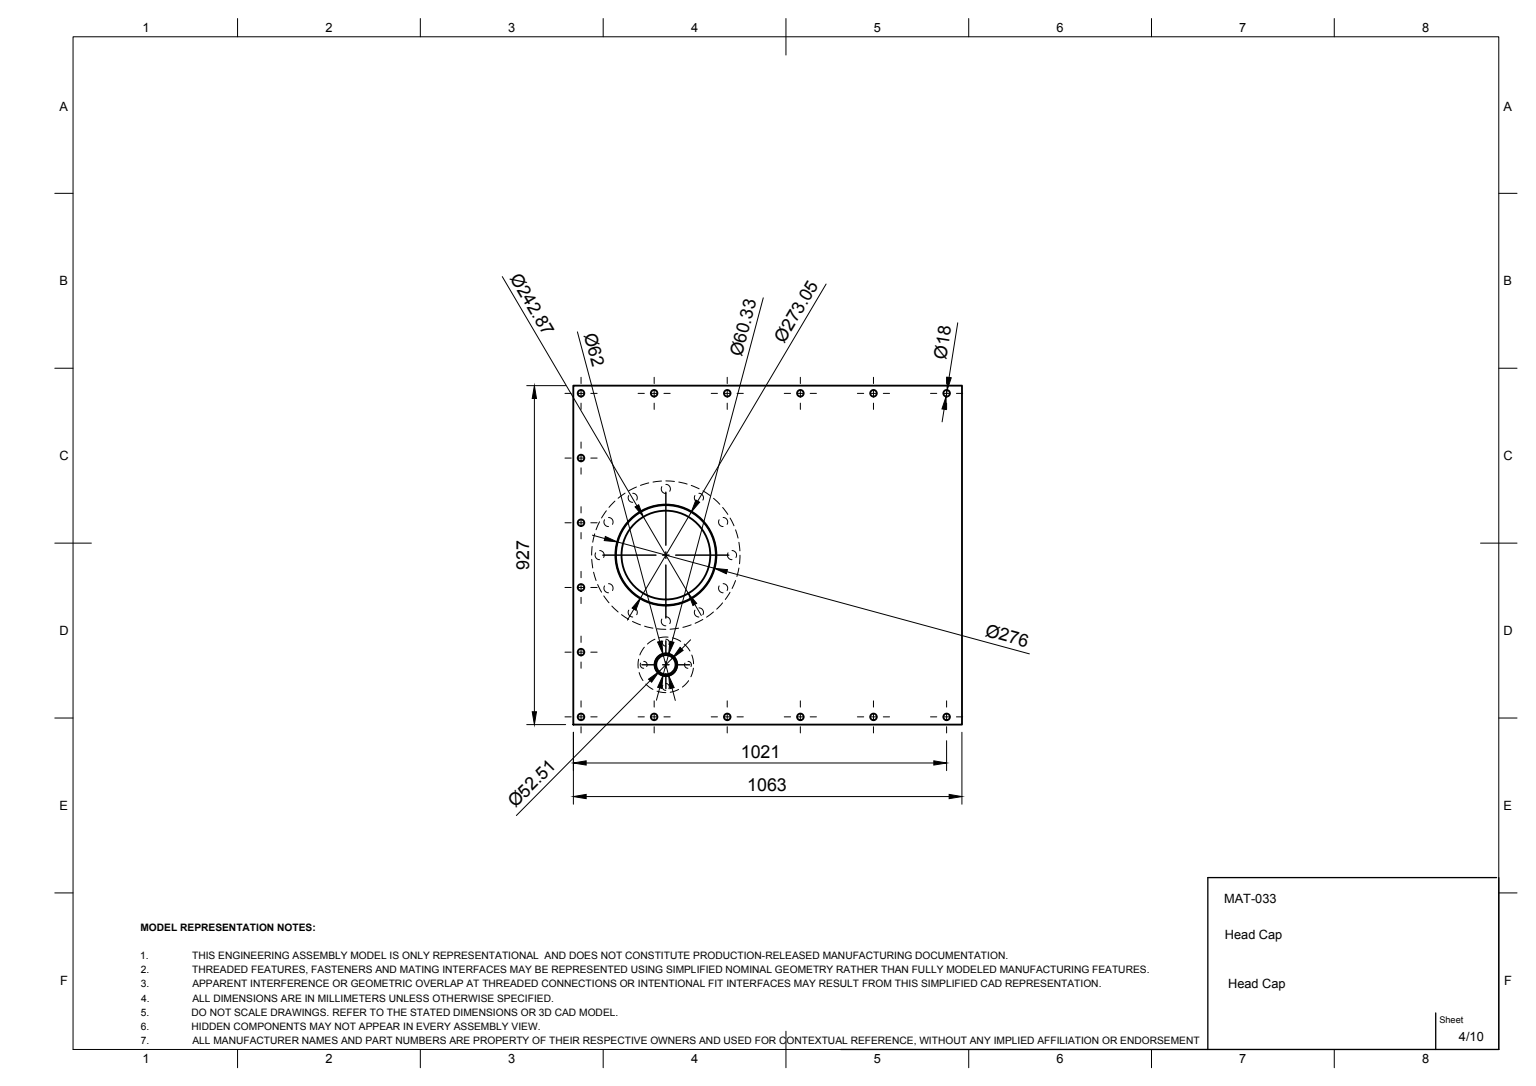
ISO-10303-21;
HEADER;
/* Generated by software containing ST-Developer
 * from STEP Tools, Inc. (www.steptools.com) 
 */

FILE_DESCRIPTION(
/* description */ ('STEP AP214'),
/* implementation_level */ '2;1');

FILE_NAME(
/* name */ 'Head Cap.step',
/* time_stamp */ '2026-11-14T07:13:32-08:00',
/* author */ (''),
/* organization */ (''),
/* preprocessor_version */ 'ST-DEVELOPER v20.2',
/* originating_system */ 'Autodesk Translation Framework v15.17.0.0',
/* authorisation */ '');

FILE_SCHEMA (('AUTOMOTIVE_DESIGN { 1 0 10303 214 3 1 1 }'));
ENDSEC;

DATA;
#10=MECHANICAL_DESIGN_GEOMETRIC_PRESENTATION_REPRESENTATION('',(#1300,#1301,#1302,#1303,#1304),#32903);
#673=SHAPE_REPRESENTATION_RELATIONSHIP('SRR','None',#33014,#687);
#687=ADVANCED_BREP_SHAPE_REPRESENTATION('',(#1389,#1390,#1391,#1392,#1393),
#32889);
#736=CIRCLE('',#15901,9.00000000000006);
#737=CIRCLE('',#15902,9.00000000000006);
#738=CIRCLE('',#15904,9.00000000000006);
#739=CIRCLE('',#15905,9.00000000000006);
#740=CIRCLE('',#15907,9.00000000000005);
#741=CIRCLE('',#15908,9.00000000000005);
#742=CIRCLE('',#15910,9.00000000000005);
#743=CIRCLE('',#15911,9.00000000000005);
#744=CIRCLE('',#15913,9.00000000000006);
#745=CIRCLE('',#15914,9.00000000000006);
#746=CIRCLE('',#15916,9.00000000000006);
#747=CIRCLE('',#15917,9.00000000000006);
#748=CIRCLE('',#15919,9.00000000000006);
#749=CIRCLE('',#15920,9.00000000000006);
#750=CIRCLE('',#15922,9.00000000000006);
#751=CIRCLE('',#15923,9.00000000000006);
#752=CIRCLE('',#15925,9.00000000000006);
#753=CIRCLE('',#15926,9.00000000000006);
#754=CIRCLE('',#15928,9.00000000000006);
#755=CIRCLE('',#15929,9.00000000000006);
#756=CIRCLE('',#15931,9.00000000000406);
#757=CIRCLE('',#15932,9.00000000000406);
#758=CIRCLE('',#15934,9.00000000000006);
#759=CIRCLE('',#15935,9.00000000000006);
#760=CIRCLE('',#15937,9.00000000000006);
#761=CIRCLE('',#15938,9.00000000000006);
#762=CIRCLE('',#15940,9.00000000000006);
#763=CIRCLE('',#15941,9.00000000000006);
#764=CIRCLE('',#15943,9.00000000000006);
#765=CIRCLE('',#15944,9.00000000000006);
#766=CIRCLE('',#15946,31.0000000000001);
#767=CIRCLE('',#15947,31.0000000000001);
#768=CIRCLE('',#15949,138.);
#769=CIRCLE('',#15950,138.);
#770=CIRCLE('',#15952,9.00000000000006);
#771=CIRCLE('',#15953,9.00000000000006);
#772=CIRCLE('',#15961,136.525);
#773=CIRCLE('',#15962,136.525);
#774=CIRCLE('',#15964,121.435);
#775=CIRCLE('',#15965,121.435);
#776=CIRCLE('',#15969,30.165);
#777=CIRCLE('',#15970,30.165);
#778=CIRCLE('',#15972,26.255);
#779=CIRCLE('',#15973,26.255);
#780=CIRCLE('',#15977,12.4999999999953);
#781=CIRCLE('',#15978,12.4999999999953);
#782=CIRCLE('',#15980,12.4999999999835);
#783=CIRCLE('',#15981,12.4999999999835);
#784=CIRCLE('',#15983,12.4999999999698);
#785=CIRCLE('',#15984,12.4999999999698);
#786=CIRCLE('',#15986,12.4999999999583);
#787=CIRCLE('',#15987,12.4999999999583);
#788=CIRCLE('',#15989,12.4999999999518);
#789=CIRCLE('',#15990,12.4999999999518);
#790=CIRCLE('',#15992,12.4999999999521);
#791=CIRCLE('',#15993,12.4999999999521);
#792=CIRCLE('',#15995,12.499999999959);
#793=CIRCLE('',#15996,12.499999999959);
#794=CIRCLE('',#15998,12.4999999999705);
#795=CIRCLE('',#15999,12.4999999999705);
#796=CIRCLE('',#16001,12.4999999999835);
#797=CIRCLE('',#16002,12.4999999999835);
#798=CIRCLE('',#16004,12.4999999999946);
#799=CIRCLE('',#16005,12.4999999999946);
#800=CIRCLE('',#16007,12.5000000000006);
#801=CIRCLE('',#16008,12.5000000000006);
#802=CIRCLE('',#16010,12.5);
#803=CIRCLE('',#16011,12.5);
#804=CIRCLE('',#16013,138.);
#805=CIRCLE('',#16014,138.);
#806=CIRCLE('',#16016,203.);
#807=CIRCLE('',#16017,203.);
#808=CIRCLE('',#16021,9.50000000000001);
#809=CIRCLE('',#16022,9.50000000000001);
#810=CIRCLE('',#16024,9.50000000000006);
#811=CIRCLE('',#16025,9.50000000000006);
#812=CIRCLE('',#16027,9.50000000000001);
#813=CIRCLE('',#16028,9.49999999999998);
#814=CIRCLE('',#16030,9.50000000000001);
#815=CIRCLE('',#16031,9.50000000000001);
#816=CIRCLE('',#16033,31.);
#817=CIRCLE('',#16034,31.);
#818=CIRCLE('',#16036,76.0000000000001);
#819=CIRCLE('',#16037,76.0000000000001);
#1099=CYLINDRICAL_SURFACE('',#15900,9.00000000000006);
#1100=CYLINDRICAL_SURFACE('',#15903,9.00000000000006);
#1101=CYLINDRICAL_SURFACE('',#15906,9.00000000000005);
#1102=CYLINDRICAL_SURFACE('',#15909,9.00000000000005);
#1103=CYLINDRICAL_SURFACE('',#15912,9.00000000000006);
#1104=CYLINDRICAL_SURFACE('',#15915,9.00000000000006);
#1105=CYLINDRICAL_SURFACE('',#15918,9.00000000000006);
#1106=CYLINDRICAL_SURFACE('',#15921,9.00000000000006);
#1107=CYLINDRICAL_SURFACE('',#15924,9.00000000000006);
#1108=CYLINDRICAL_SURFACE('',#15927,9.00000000000006);
#1109=CYLINDRICAL_SURFACE('',#15930,9.00000000000406);
#1110=CYLINDRICAL_SURFACE('',#15933,9.00000000000006);
#1111=CYLINDRICAL_SURFACE('',#15936,9.00000000000006);
#1112=CYLINDRICAL_SURFACE('',#15939,9.00000000000006);
#1113=CYLINDRICAL_SURFACE('',#15942,9.00000000000006);
#1114=CYLINDRICAL_SURFACE('',#15945,31.0000000000001);
#1115=CYLINDRICAL_SURFACE('',#15948,138.);
#1116=CYLINDRICAL_SURFACE('',#15951,9.00000000000006);
#1117=CYLINDRICAL_SURFACE('',#15960,136.525);
#1118=CYLINDRICAL_SURFACE('',#15963,121.435);
#1119=CYLINDRICAL_SURFACE('',#15968,30.165);
#1120=CYLINDRICAL_SURFACE('',#15971,26.255);
#1121=CYLINDRICAL_SURFACE('',#15976,12.4999999999953);
#1122=CYLINDRICAL_SURFACE('',#15979,12.4999999999835);
#1123=CYLINDRICAL_SURFACE('',#15982,12.4999999999698);
#1124=CYLINDRICAL_SURFACE('',#15985,12.4999999999583);
#1125=CYLINDRICAL_SURFACE('',#15988,12.4999999999518);
#1126=CYLINDRICAL_SURFACE('',#15991,12.4999999999521);
#1127=CYLINDRICAL_SURFACE('',#15994,12.499999999959);
#1128=CYLINDRICAL_SURFACE('',#15997,12.4999999999705);
#1129=CYLINDRICAL_SURFACE('',#16000,12.4999999999835);
#1130=CYLINDRICAL_SURFACE('',#16003,12.4999999999946);
#1131=CYLINDRICAL_SURFACE('',#16006,12.5000000000006);
#1132=CYLINDRICAL_SURFACE('',#16009,12.5);
#1133=CYLINDRICAL_SURFACE('',#16012,138.);
#1134=CYLINDRICAL_SURFACE('',#16015,203.);
#1135=CYLINDRICAL_SURFACE('',#16020,9.50000000000001);
#1136=CYLINDRICAL_SURFACE('',#16023,9.50000000000006);
#1137=CYLINDRICAL_SURFACE('',#16026,9.50000000000001);
#1138=CYLINDRICAL_SURFACE('',#16029,9.50000000000001);
#1139=CYLINDRICAL_SURFACE('',#16032,31.);
#1140=CYLINDRICAL_SURFACE('',#16035,76.0000000000001);
#1300=STYLED_ITEM('',(#33097),#1389);
#1301=STYLED_ITEM('',(#33097),#1390);
#1302=STYLED_ITEM('',(#33097),#1391);
#1303=STYLED_ITEM('',(#33097),#1392);
#1304=STYLED_ITEM('',(#33097),#1393);
#1389=MANIFOLD_SOLID_BREP('Body1',#15548);
#1390=MANIFOLD_SOLID_BREP('Body2',#15549);
#1391=MANIFOLD_SOLID_BREP('Body3',#15550);
#1392=MANIFOLD_SOLID_BREP('Body4',#15551);
#1393=MANIFOLD_SOLID_BREP('Body5',#15552);
#1503=FACE_BOUND('',#2706,.T.);
#1504=FACE_BOUND('',#2707,.T.);
#1505=FACE_BOUND('',#2708,.T.);
#1506=FACE_BOUND('',#2709,.T.);
#1507=FACE_BOUND('',#2710,.T.);
#1508=FACE_BOUND('',#2711,.T.);
#1509=FACE_BOUND('',#2712,.T.);
#1510=FACE_BOUND('',#2713,.T.);
#1511=FACE_BOUND('',#2714,.T.);
#1512=FACE_BOUND('',#2715,.T.);
#1513=FACE_BOUND('',#2716,.T.);
#1514=FACE_BOUND('',#2717,.T.);
#1515=FACE_BOUND('',#2718,.T.);
#1516=FACE_BOUND('',#2719,.T.);
#1517=FACE_BOUND('',#2720,.T.);
#1518=FACE_BOUND('',#2721,.T.);
#1519=FACE_BOUND('',#2722,.T.);
#1520=FACE_BOUND('',#2723,.T.);
#1521=FACE_BOUND('',#2725,.T.);
#1522=FACE_BOUND('',#2726,.T.);
#1523=FACE_BOUND('',#2727,.T.);
#1524=FACE_BOUND('',#2728,.T.);
#1525=FACE_BOUND('',#2729,.T.);
#1526=FACE_BOUND('',#2730,.T.);
#1527=FACE_BOUND('',#2731,.T.);
#1528=FACE_BOUND('',#2732,.T.);
#1529=FACE_BOUND('',#2733,.T.);
#1530=FACE_BOUND('',#2734,.T.);
#1531=FACE_BOUND('',#2735,.T.);
#1532=FACE_BOUND('',#2736,.T.);
#1533=FACE_BOUND('',#2737,.T.);
#1534=FACE_BOUND('',#2738,.T.);
#1535=FACE_BOUND('',#2739,.T.);
#1536=FACE_BOUND('',#2740,.T.);
#1537=FACE_BOUND('',#2741,.T.);
#1538=FACE_BOUND('',#2742,.T.);
#1539=FACE_BOUND('',#2746,.T.);
#1540=FACE_BOUND('',#2748,.T.);
#1541=FACE_BOUND('',#2752,.T.);
#1542=FACE_BOUND('',#2754,.T.);
#1543=FACE_BOUND('',#2770,.T.);
#1544=FACE_BOUND('',#2771,.T.);
#1545=FACE_BOUND('',#2772,.T.);
#1546=FACE_BOUND('',#2773,.T.);
#1547=FACE_BOUND('',#2774,.T.);
#1548=FACE_BOUND('',#2775,.T.);
#1549=FACE_BOUND('',#2776,.T.);
#1550=FACE_BOUND('',#2777,.T.);
#1551=FACE_BOUND('',#2778,.T.);
#1552=FACE_BOUND('',#2779,.T.);
#1553=FACE_BOUND('',#2780,.T.);
#1554=FACE_BOUND('',#2781,.T.);
#1555=FACE_BOUND('',#2782,.T.);
#1556=FACE_BOUND('',#2784,.T.);
#1557=FACE_BOUND('',#2785,.T.);
#1558=FACE_BOUND('',#2786,.T.);
#1559=FACE_BOUND('',#2787,.T.);
#1560=FACE_BOUND('',#2788,.T.);
#1561=FACE_BOUND('',#2789,.T.);
#1562=FACE_BOUND('',#2790,.T.);
#1563=FACE_BOUND('',#2791,.T.);
#1564=FACE_BOUND('',#2792,.T.);
#1565=FACE_BOUND('',#2793,.T.);
#1566=FACE_BOUND('',#2794,.T.);
#1567=FACE_BOUND('',#2795,.T.);
#1568=FACE_BOUND('',#2796,.T.);
#1569=FACE_BOUND('',#2804,.T.);
#1570=FACE_BOUND('',#2805,.T.);
#1571=FACE_BOUND('',#2806,.T.);
#1572=FACE_BOUND('',#2807,.T.);
#1573=FACE_BOUND('',#2808,.T.);
#1574=FACE_BOUND('',#2810,.T.);
#1575=FACE_BOUND('',#2811,.T.);
#1576=FACE_BOUND('',#2812,.T.);
#1577=FACE_BOUND('',#2813,.T.);
#1578=FACE_BOUND('',#2814,.T.);
#1754=FACE_OUTER_BOUND('',#2683,.T.);
#1755=FACE_OUTER_BOUND('',#2684,.T.);
#1756=FACE_OUTER_BOUND('',#2685,.T.);
#1757=FACE_OUTER_BOUND('',#2686,.T.);
#1758=FACE_OUTER_BOUND('',#2687,.T.);
#1759=FACE_OUTER_BOUND('',#2688,.T.);
#1760=FACE_OUTER_BOUND('',#2689,.T.);
#1761=FACE_OUTER_BOUND('',#2690,.T.);
#1762=FACE_OUTER_BOUND('',#2691,.T.);
#1763=FACE_OUTER_BOUND('',#2692,.T.);
#1764=FACE_OUTER_BOUND('',#2693,.T.);
#1765=FACE_OUTER_BOUND('',#2694,.T.);
#1766=FACE_OUTER_BOUND('',#2695,.T.);
#1767=FACE_OUTER_BOUND('',#2696,.T.);
#1768=FACE_OUTER_BOUND('',#2697,.T.);
#1769=FACE_OUTER_BOUND('',#2698,.T.);
#1770=FACE_OUTER_BOUND('',#2699,.T.);
#1771=FACE_OUTER_BOUND('',#2700,.T.);
#1772=FACE_OUTER_BOUND('',#2701,.T.);
#1773=FACE_OUTER_BOUND('',#2702,.T.);
#1774=FACE_OUTER_BOUND('',#2703,.T.);
#1775=FACE_OUTER_BOUND('',#2704,.T.);
#1776=FACE_OUTER_BOUND('',#2705,.T.);
#1777=FACE_OUTER_BOUND('',#2724,.T.);
#1778=FACE_OUTER_BOUND('',#2743,.T.);
#1779=FACE_OUTER_BOUND('',#2744,.T.);
#1780=FACE_OUTER_BOUND('',#2745,.T.);
#1781=FACE_OUTER_BOUND('',#2747,.T.);
#1782=FACE_OUTER_BOUND('',#2749,.T.);
#1783=FACE_OUTER_BOUND('',#2750,.T.);
#1784=FACE_OUTER_BOUND('',#2751,.T.);
#1785=FACE_OUTER_BOUND('',#2753,.T.);
#1786=FACE_OUTER_BOUND('',#2755,.T.);
#1787=FACE_OUTER_BOUND('',#2756,.T.);
#1788=FACE_OUTER_BOUND('',#2757,.T.);
#1789=FACE_OUTER_BOUND('',#2758,.T.);
#1790=FACE_OUTER_BOUND('',#2759,.T.);
#1791=FACE_OUTER_BOUND('',#2760,.T.);
#1792=FACE_OUTER_BOUND('',#2761,.T.);
#1793=FACE_OUTER_BOUND('',#2762,.T.);
#1794=FACE_OUTER_BOUND('',#2763,.T.);
#1795=FACE_OUTER_BOUND('',#2764,.T.);
#1796=FACE_OUTER_BOUND('',#2765,.T.);
#1797=FACE_OUTER_BOUND('',#2766,.T.);
#1798=FACE_OUTER_BOUND('',#2767,.T.);
#1799=FACE_OUTER_BOUND('',#2768,.T.);
#1800=FACE_OUTER_BOUND('',#2769,.T.);
#1801=FACE_OUTER_BOUND('',#2783,.T.);
#1802=FACE_OUTER_BOUND('',#2797,.T.);
#1803=FACE_OUTER_BOUND('',#2798,.T.);
#1804=FACE_OUTER_BOUND('',#2799,.T.);
#1805=FACE_OUTER_BOUND('',#2800,.T.);
#1806=FACE_OUTER_BOUND('',#2801,.T.);
#1807=FACE_OUTER_BOUND('',#2802,.T.);
#1808=FACE_OUTER_BOUND('',#2803,.T.);
#1809=FACE_OUTER_BOUND('',#2809,.T.);
#2683=EDGE_LOOP('',(#10267,#10268,#10269,#10270));
#2684=EDGE_LOOP('',(#10271,#10272,#10273,#10274));
#2685=EDGE_LOOP('',(#10275,#10276,#10277,#10278));
#2686=EDGE_LOOP('',(#10279,#10280,#10281,#10282));
#2687=EDGE_LOOP('',(#10283,#10284,#10285,#10286));
#2688=EDGE_LOOP('',(#10287,#10288,#10289,#10290));
#2689=EDGE_LOOP('',(#10291,#10292,#10293,#10294));
#2690=EDGE_LOOP('',(#10295,#10296,#10297,#10298));
#2691=EDGE_LOOP('',(#10299,#10300,#10301,#10302));
#2692=EDGE_LOOP('',(#10303,#10304,#10305,#10306));
#2693=EDGE_LOOP('',(#10307,#10308,#10309,#10310));
#2694=EDGE_LOOP('',(#10311,#10312,#10313,#10314));
#2695=EDGE_LOOP('',(#10315,#10316,#10317,#10318));
#2696=EDGE_LOOP('',(#10319,#10320,#10321,#10322));
#2697=EDGE_LOOP('',(#10323,#10324,#10325,#10326));
#2698=EDGE_LOOP('',(#10327,#10328,#10329,#10330));
#2699=EDGE_LOOP('',(#10331,#10332,#10333,#10334));
#2700=EDGE_LOOP('',(#10335,#10336,#10337,#10338));
#2701=EDGE_LOOP('',(#10339,#10340,#10341,#10342));
#2702=EDGE_LOOP('',(#10343,#10344,#10345,#10346));
#2703=EDGE_LOOP('',(#10347,#10348,#10349,#10350));
#2704=EDGE_LOOP('',(#10351,#10352,#10353,#10354));
#2705=EDGE_LOOP('',(#10355,#10356,#10357,#10358));
#2706=EDGE_LOOP('',(#10359));
#2707=EDGE_LOOP('',(#10360));
#2708=EDGE_LOOP('',(#10361));
#2709=EDGE_LOOP('',(#10362));
#2710=EDGE_LOOP('',(#10363));
#2711=EDGE_LOOP('',(#10364));
#2712=EDGE_LOOP('',(#10365));
#2713=EDGE_LOOP('',(#10366));
#2714=EDGE_LOOP('',(#10367));
#2715=EDGE_LOOP('',(#10368));
#2716=EDGE_LOOP('',(#10369));
#2717=EDGE_LOOP('',(#10370));
#2718=EDGE_LOOP('',(#10371));
#2719=EDGE_LOOP('',(#10372));
#2720=EDGE_LOOP('',(#10373));
#2721=EDGE_LOOP('',(#10374));
#2722=EDGE_LOOP('',(#10375));
#2723=EDGE_LOOP('',(#10376));
#2724=EDGE_LOOP('',(#10377,#10378,#10379,#10380));
#2725=EDGE_LOOP('',(#10381));
#2726=EDGE_LOOP('',(#10382));
#2727=EDGE_LOOP('',(#10383));
#2728=EDGE_LOOP('',(#10384));
#2729=EDGE_LOOP('',(#10385));
#2730=EDGE_LOOP('',(#10386));
#2731=EDGE_LOOP('',(#10387));
#2732=EDGE_LOOP('',(#10388));
#2733=EDGE_LOOP('',(#10389));
#2734=EDGE_LOOP('',(#10390));
#2735=EDGE_LOOP('',(#10391));
#2736=EDGE_LOOP('',(#10392));
#2737=EDGE_LOOP('',(#10393));
#2738=EDGE_LOOP('',(#10394));
#2739=EDGE_LOOP('',(#10395));
#2740=EDGE_LOOP('',(#10396));
#2741=EDGE_LOOP('',(#10397));
#2742=EDGE_LOOP('',(#10398));
#2743=EDGE_LOOP('',(#10399,#10400,#10401,#10402));
#2744=EDGE_LOOP('',(#10403,#10404,#10405,#10406));
#2745=EDGE_LOOP('',(#10407));
#2746=EDGE_LOOP('',(#10408));
#2747=EDGE_LOOP('',(#10409));
#2748=EDGE_LOOP('',(#10410));
#2749=EDGE_LOOP('',(#10411,#10412,#10413,#10414));
#2750=EDGE_LOOP('',(#10415,#10416,#10417,#10418));
#2751=EDGE_LOOP('',(#10419));
#2752=EDGE_LOOP('',(#10420));
#2753=EDGE_LOOP('',(#10421));
#2754=EDGE_LOOP('',(#10422));
#2755=EDGE_LOOP('',(#10423,#10424,#10425,#10426));
#2756=EDGE_LOOP('',(#10427,#10428,#10429,#10430));
#2757=EDGE_LOOP('',(#10431,#10432,#10433,#10434));
#2758=EDGE_LOOP('',(#10435,#10436,#10437,#10438));
#2759=EDGE_LOOP('',(#10439,#10440,#10441,#10442));
#2760=EDGE_LOOP('',(#10443,#10444,#10445,#10446));
#2761=EDGE_LOOP('',(#10447,#10448,#10449,#10450));
#2762=EDGE_LOOP('',(#10451,#10452,#10453,#10454));
#2763=EDGE_LOOP('',(#10455,#10456,#10457,#10458));
#2764=EDGE_LOOP('',(#10459,#10460,#10461,#10462));
#2765=EDGE_LOOP('',(#10463,#10464,#10465,#10466));
#2766=EDGE_LOOP('',(#10467,#10468,#10469,#10470));
#2767=EDGE_LOOP('',(#10471,#10472,#10473,#10474));
#2768=EDGE_LOOP('',(#10475,#10476,#10477,#10478));
#2769=EDGE_LOOP('',(#10479));
#2770=EDGE_LOOP('',(#10480));
#2771=EDGE_LOOP('',(#10481));
#2772=EDGE_LOOP('',(#10482));
#2773=EDGE_LOOP('',(#10483));
#2774=EDGE_LOOP('',(#10484));
#2775=EDGE_LOOP('',(#10485));
#2776=EDGE_LOOP('',(#10486));
#2777=EDGE_LOOP('',(#10487));
#2778=EDGE_LOOP('',(#10488));
#2779=EDGE_LOOP('',(#10489));
#2780=EDGE_LOOP('',(#10490));
#2781=EDGE_LOOP('',(#10491));
#2782=EDGE_LOOP('',(#10492));
#2783=EDGE_LOOP('',(#10493));
#2784=EDGE_LOOP('',(#10494));
#2785=EDGE_LOOP('',(#10495));
#2786=EDGE_LOOP('',(#10496));
#2787=EDGE_LOOP('',(#10497));
#2788=EDGE_LOOP('',(#10498));
#2789=EDGE_LOOP('',(#10499));
#2790=EDGE_LOOP('',(#10500));
#2791=EDGE_LOOP('',(#10501));
#2792=EDGE_LOOP('',(#10502));
#2793=EDGE_LOOP('',(#10503));
#2794=EDGE_LOOP('',(#10504));
#2795=EDGE_LOOP('',(#10505));
#2796=EDGE_LOOP('',(#10506));
#2797=EDGE_LOOP('',(#10507,#10508,#10509,#10510));
#2798=EDGE_LOOP('',(#10511,#10512,#10513,#10514));
#2799=EDGE_LOOP('',(#10515,#10516,#10517,#10518));
#2800=EDGE_LOOP('',(#10519,#10520,#10521,#10522));
#2801=EDGE_LOOP('',(#10523,#10524,#10525,#10526));
#2802=EDGE_LOOP('',(#10527,#10528,#10529,#10530));
#2803=EDGE_LOOP('',(#10531));
#2804=EDGE_LOOP('',(#10532));
#2805=EDGE_LOOP('',(#10533));
#2806=EDGE_LOOP('',(#10534));
#2807=EDGE_LOOP('',(#10535));
#2808=EDGE_LOOP('',(#10536));
#2809=EDGE_LOOP('',(#10537));
#2810=EDGE_LOOP('',(#10538));
#2811=EDGE_LOOP('',(#10539));
#2812=EDGE_LOOP('',(#10540));
#2813=EDGE_LOOP('',(#10541));
#2814=EDGE_LOOP('',(#10542));
#3817=LINE('',#21694,#5221);
#3818=LINE('',#21700,#5222);
#3819=LINE('',#21706,#5223);
#3820=LINE('',#21712,#5224);
#3821=LINE('',#21718,#5225);
#3822=LINE('',#21724,#5226);
#3823=LINE('',#21730,#5227);
#3824=LINE('',#21736,#5228);
#3825=LINE('',#21742,#5229);
#3826=LINE('',#21748,#5230);
#3827=LINE('',#21754,#5231);
#3828=LINE('',#21760,#5232);
#3829=LINE('',#21766,#5233);
#3830=LINE('',#21772,#5234);
#3831=LINE('',#21778,#5235);
#3832=LINE('',#21784,#5236);
#3833=LINE('',#21790,#5237);
#3834=LINE('',#21796,#5238);
#3835=LINE('',#21801,#5239);
#3836=LINE('',#21803,#5240);
#3837=LINE('',#21805,#5241);
#3838=LINE('',#21806,#5242);
#3839=LINE('',#21809,#5243);
#3840=LINE('',#21811,#5244);
#3841=LINE('',#21812,#5245);
#3842=LINE('',#21815,#5246);
#3843=LINE('',#21817,#5247);
#3844=LINE('',#21818,#5248);
#3845=LINE('',#21820,#5249);
#3846=LINE('',#21821,#5250);
#3847=LINE('',#21828,#5251);
#3848=LINE('',#21834,#5252);
#3849=LINE('',#21842,#5253);
#3850=LINE('',#21848,#5254);
#3851=LINE('',#21856,#5255);
#3852=LINE('',#21862,#5256);
#3853=LINE('',#21868,#5257);
#3854=LINE('',#21874,#5258);
#3855=LINE('',#21880,#5259);
#3856=LINE('',#21886,#5260);
#3857=LINE('',#21892,#5261);
#3858=LINE('',#21898,#5262);
#3859=LINE('',#21904,#5263);
#3860=LINE('',#21910,#5264);
#3861=LINE('',#21916,#5265);
#3862=LINE('',#21922,#5266);
#3863=LINE('',#21928,#5267);
#3864=LINE('',#21934,#5268);
#3865=LINE('',#21942,#5269);
#3866=LINE('',#21948,#5270);
#3867=LINE('',#21954,#5271);
#3868=LINE('',#21960,#5272);
#3869=LINE('',#21966,#5273);
#3870=LINE('',#21972,#5274);
#5221=VECTOR('',#17539,9.00000000000006);
#5222=VECTOR('',#17546,9.00000000000006);
#5223=VECTOR('',#17553,9.00000000000005);
#5224=VECTOR('',#17560,9.00000000000005);
#5225=VECTOR('',#17567,9.00000000000006);
#5226=VECTOR('',#17574,9.00000000000006);
#5227=VECTOR('',#17581,9.00000000000006);
#5228=VECTOR('',#17588,9.00000000000006);
#5229=VECTOR('',#17595,9.00000000000006);
#5230=VECTOR('',#17602,9.00000000000006);
#5231=VECTOR('',#17609,9.00000000000406);
#5232=VECTOR('',#17616,9.00000000000006);
#5233=VECTOR('',#17623,9.00000000000006);
#5234=VECTOR('',#17630,9.00000000000006);
#5235=VECTOR('',#17637,9.00000000000006);
#5236=VECTOR('',#17644,31.0000000000001);
#5237=VECTOR('',#17651,138.);
#5238=VECTOR('',#17658,9.00000000000006);
#5239=VECTOR('',#17663,1000.);
#5240=VECTOR('',#17664,1000.);
#5241=VECTOR('',#17665,1000.);
#5242=VECTOR('',#17666,1000.);
#5243=VECTOR('',#17669,1000.);
#5244=VECTOR('',#17670,1000.);
#5245=VECTOR('',#17671,1000.);
#5246=VECTOR('',#17674,1000.);
#5247=VECTOR('',#17675,1000.);
#5248=VECTOR('',#17676,1000.);
#5249=VECTOR('',#17679,1000.);
#5250=VECTOR('',#17680,1000.);
#5251=VECTOR('',#17689,136.525);
#5252=VECTOR('',#17696,121.435);
#5253=VECTOR('',#17707,30.165);
#5254=VECTOR('',#17714,26.255);
#5255=VECTOR('',#17725,12.4999999999953);
#5256=VECTOR('',#17732,12.4999999999835);
#5257=VECTOR('',#17739,12.4999999999698);
#5258=VECTOR('',#17746,12.4999999999583);
#5259=VECTOR('',#17753,12.4999999999518);
#5260=VECTOR('',#17760,12.4999999999521);
#5261=VECTOR('',#17767,12.499999999959);
#5262=VECTOR('',#17774,12.4999999999705);
#5263=VECTOR('',#17781,12.4999999999835);
#5264=VECTOR('',#17788,12.4999999999946);
#5265=VECTOR('',#17795,12.5000000000006);
#5266=VECTOR('',#17802,12.5);
#5267=VECTOR('',#17809,138.);
#5268=VECTOR('',#17816,203.);
#5269=VECTOR('',#17827,9.50000000000001);
#5270=VECTOR('',#17834,9.50000000000006);
#5271=VECTOR('',#17841,9.50000000000001);
#5272=VECTOR('',#17848,9.50000000000001);
#5273=VECTOR('',#17855,31.);
#5274=VECTOR('',#17862,76.0000000000001);
#6601=VERTEX_POINT('',#21691);
#6602=VERTEX_POINT('',#21693);
#6603=VERTEX_POINT('',#21697);
#6604=VERTEX_POINT('',#21699);
#6605=VERTEX_POINT('',#21703);
#6606=VERTEX_POINT('',#21705);
#6607=VERTEX_POINT('',#21709);
#6608=VERTEX_POINT('',#21711);
#6609=VERTEX_POINT('',#21715);
#6610=VERTEX_POINT('',#21717);
#6611=VERTEX_POINT('',#21721);
#6612=VERTEX_POINT('',#21723);
#6613=VERTEX_POINT('',#21727);
#6614=VERTEX_POINT('',#21729);
#6615=VERTEX_POINT('',#21733);
#6616=VERTEX_POINT('',#21735);
#6617=VERTEX_POINT('',#21739);
#6618=VERTEX_POINT('',#21741);
#6619=VERTEX_POINT('',#21745);
#6620=VERTEX_POINT('',#21747);
#6621=VERTEX_POINT('',#21751);
#6622=VERTEX_POINT('',#21753);
#6623=VERTEX_POINT('',#21757);
#6624=VERTEX_POINT('',#21759);
#6625=VERTEX_POINT('',#21763);
#6626=VERTEX_POINT('',#21765);
#6627=VERTEX_POINT('',#21769);
#6628=VERTEX_POINT('',#21771);
#6629=VERTEX_POINT('',#21775);
#6630=VERTEX_POINT('',#21777);
#6631=VERTEX_POINT('',#21781);
#6632=VERTEX_POINT('',#21783);
#6633=VERTEX_POINT('',#21787);
#6634=VERTEX_POINT('',#21789);
#6635=VERTEX_POINT('',#21793);
#6636=VERTEX_POINT('',#21795);
#6637=VERTEX_POINT('',#21799);
#6638=VERTEX_POINT('',#21800);
#6639=VERTEX_POINT('',#21802);
#6640=VERTEX_POINT('',#21804);
#6641=VERTEX_POINT('',#21808);
#6642=VERTEX_POINT('',#21810);
#6643=VERTEX_POINT('',#21814);
#6644=VERTEX_POINT('',#21816);
#6645=VERTEX_POINT('',#21825);
#6646=VERTEX_POINT('',#21827);
#6647=VERTEX_POINT('',#21831);
#6648=VERTEX_POINT('',#21833);
#6649=VERTEX_POINT('',#21839);
#6650=VERTEX_POINT('',#21841);
#6651=VERTEX_POINT('',#21845);
#6652=VERTEX_POINT('',#21847);
#6653=VERTEX_POINT('',#21853);
#6654=VERTEX_POINT('',#21855);
#6655=VERTEX_POINT('',#21859);
#6656=VERTEX_POINT('',#21861);
#6657=VERTEX_POINT('',#21865);
#6658=VERTEX_POINT('',#21867);
#6659=VERTEX_POINT('',#21871);
#6660=VERTEX_POINT('',#21873);
#6661=VERTEX_POINT('',#21877);
#6662=VERTEX_POINT('',#21879);
#6663=VERTEX_POINT('',#21883);
#6664=VERTEX_POINT('',#21885);
#6665=VERTEX_POINT('',#21889);
#6666=VERTEX_POINT('',#21891);
#6667=VERTEX_POINT('',#21895);
#6668=VERTEX_POINT('',#21897);
#6669=VERTEX_POINT('',#21901);
#6670=VERTEX_POINT('',#21903);
#6671=VERTEX_POINT('',#21907);
#6672=VERTEX_POINT('',#21909);
#6673=VERTEX_POINT('',#21913);
#6674=VERTEX_POINT('',#21915);
#6675=VERTEX_POINT('',#21919);
#6676=VERTEX_POINT('',#21921);
#6677=VERTEX_POINT('',#21925);
#6678=VERTEX_POINT('',#21927);
#6679=VERTEX_POINT('',#21931);
#6680=VERTEX_POINT('',#21933);
#6681=VERTEX_POINT('',#21939);
#6682=VERTEX_POINT('',#21941);
#6683=VERTEX_POINT('',#21945);
#6684=VERTEX_POINT('',#21947);
#6685=VERTEX_POINT('',#21951);
#6686=VERTEX_POINT('',#21953);
#6687=VERTEX_POINT('',#21957);
#6688=VERTEX_POINT('',#21959);
#6689=VERTEX_POINT('',#21963);
#6690=VERTEX_POINT('',#21965);
#6691=VERTEX_POINT('',#21969);
#6692=VERTEX_POINT('',#21971);
#8017=EDGE_CURVE('',#6601,#6601,#736,.T.);
#8018=EDGE_CURVE('',#6601,#6602,#3817,.T.);
#8019=EDGE_CURVE('',#6602,#6602,#737,.T.);
#8020=EDGE_CURVE('',#6603,#6603,#738,.T.);
#8021=EDGE_CURVE('',#6603,#6604,#3818,.T.);
#8022=EDGE_CURVE('',#6604,#6604,#739,.T.);
#8023=EDGE_CURVE('',#6605,#6605,#740,.T.);
#8024=EDGE_CURVE('',#6605,#6606,#3819,.T.);
#8025=EDGE_CURVE('',#6606,#6606,#741,.T.);
#8026=EDGE_CURVE('',#6607,#6607,#742,.T.);
#8027=EDGE_CURVE('',#6607,#6608,#3820,.T.);
#8028=EDGE_CURVE('',#6608,#6608,#743,.T.);
#8029=EDGE_CURVE('',#6609,#6609,#744,.T.);
#8030=EDGE_CURVE('',#6609,#6610,#3821,.T.);
#8031=EDGE_CURVE('',#6610,#6610,#745,.T.);
#8032=EDGE_CURVE('',#6611,#6611,#746,.T.);
#8033=EDGE_CURVE('',#6611,#6612,#3822,.T.);
#8034=EDGE_CURVE('',#6612,#6612,#747,.T.);
#8035=EDGE_CURVE('',#6613,#6613,#748,.T.);
#8036=EDGE_CURVE('',#6613,#6614,#3823,.T.);
#8037=EDGE_CURVE('',#6614,#6614,#749,.T.);
#8038=EDGE_CURVE('',#6615,#6615,#750,.T.);
#8039=EDGE_CURVE('',#6615,#6616,#3824,.T.);
#8040=EDGE_CURVE('',#6616,#6616,#751,.T.);
#8041=EDGE_CURVE('',#6617,#6617,#752,.T.);
#8042=EDGE_CURVE('',#6617,#6618,#3825,.T.);
#8043=EDGE_CURVE('',#6618,#6618,#753,.T.);
#8044=EDGE_CURVE('',#6619,#6619,#754,.T.);
#8045=EDGE_CURVE('',#6619,#6620,#3826,.T.);
#8046=EDGE_CURVE('',#6620,#6620,#755,.T.);
#8047=EDGE_CURVE('',#6621,#6621,#756,.T.);
#8048=EDGE_CURVE('',#6621,#6622,#3827,.T.);
#8049=EDGE_CURVE('',#6622,#6622,#757,.T.);
#8050=EDGE_CURVE('',#6623,#6623,#758,.T.);
#8051=EDGE_CURVE('',#6623,#6624,#3828,.T.);
#8052=EDGE_CURVE('',#6624,#6624,#759,.T.);
#8053=EDGE_CURVE('',#6625,#6625,#760,.T.);
#8054=EDGE_CURVE('',#6625,#6626,#3829,.T.);
#8055=EDGE_CURVE('',#6626,#6626,#761,.T.);
#8056=EDGE_CURVE('',#6627,#6627,#762,.T.);
#8057=EDGE_CURVE('',#6627,#6628,#3830,.T.);
#8058=EDGE_CURVE('',#6628,#6628,#763,.T.);
#8059=EDGE_CURVE('',#6629,#6629,#764,.T.);
#8060=EDGE_CURVE('',#6629,#6630,#3831,.T.);
#8061=EDGE_CURVE('',#6630,#6630,#765,.T.);
#8062=EDGE_CURVE('',#6631,#6631,#766,.T.);
#8063=EDGE_CURVE('',#6631,#6632,#3832,.T.);
#8064=EDGE_CURVE('',#6632,#6632,#767,.T.);
#8065=EDGE_CURVE('',#6633,#6633,#768,.T.);
#8066=EDGE_CURVE('',#6633,#6634,#3833,.T.);
#8067=EDGE_CURVE('',#6634,#6634,#769,.T.);
#8068=EDGE_CURVE('',#6635,#6635,#770,.T.);
#8069=EDGE_CURVE('',#6635,#6636,#3834,.T.);
#8070=EDGE_CURVE('',#6636,#6636,#771,.T.);
#8071=EDGE_CURVE('',#6637,#6638,#3835,.T.);
#8072=EDGE_CURVE('',#6639,#6637,#3836,.T.);
#8073=EDGE_CURVE('',#6639,#6640,#3837,.T.);
#8074=EDGE_CURVE('',#6640,#6638,#3838,.T.);
#8075=EDGE_CURVE('',#6641,#6637,#3839,.T.);
#8076=EDGE_CURVE('',#6642,#6641,#3840,.T.);
#8077=EDGE_CURVE('',#6642,#6639,#3841,.T.);
#8078=EDGE_CURVE('',#6643,#6641,#3842,.T.);
#8079=EDGE_CURVE('',#6644,#6643,#3843,.T.);
#8080=EDGE_CURVE('',#6644,#6642,#3844,.T.);
#8081=EDGE_CURVE('',#6638,#6643,#3845,.T.);
#8082=EDGE_CURVE('',#6640,#6644,#3846,.T.);
#8083=EDGE_CURVE('',#6645,#6645,#772,.T.);
#8084=EDGE_CURVE('',#6645,#6646,#3847,.T.);
#8085=EDGE_CURVE('',#6646,#6646,#773,.T.);
#8086=EDGE_CURVE('',#6647,#6647,#774,.T.);
#8087=EDGE_CURVE('',#6647,#6648,#3848,.T.);
#8088=EDGE_CURVE('',#6648,#6648,#775,.T.);
#8089=EDGE_CURVE('',#6649,#6649,#776,.T.);
#8090=EDGE_CURVE('',#6649,#6650,#3849,.T.);
#8091=EDGE_CURVE('',#6650,#6650,#777,.T.);
#8092=EDGE_CURVE('',#6651,#6651,#778,.T.);
#8093=EDGE_CURVE('',#6651,#6652,#3850,.T.);
#8094=EDGE_CURVE('',#6652,#6652,#779,.T.);
#8095=EDGE_CURVE('',#6653,#6653,#780,.T.);
#8096=EDGE_CURVE('',#6653,#6654,#3851,.T.);
#8097=EDGE_CURVE('',#6654,#6654,#781,.T.);
#8098=EDGE_CURVE('',#6655,#6655,#782,.T.);
#8099=EDGE_CURVE('',#6655,#6656,#3852,.T.);
#8100=EDGE_CURVE('',#6656,#6656,#783,.T.);
#8101=EDGE_CURVE('',#6657,#6657,#784,.T.);
#8102=EDGE_CURVE('',#6657,#6658,#3853,.T.);
#8103=EDGE_CURVE('',#6658,#6658,#785,.T.);
#8104=EDGE_CURVE('',#6659,#6659,#786,.T.);
#8105=EDGE_CURVE('',#6659,#6660,#3854,.T.);
#8106=EDGE_CURVE('',#6660,#6660,#787,.T.);
#8107=EDGE_CURVE('',#6661,#6661,#788,.T.);
#8108=EDGE_CURVE('',#6661,#6662,#3855,.T.);
#8109=EDGE_CURVE('',#6662,#6662,#789,.T.);
#8110=EDGE_CURVE('',#6663,#6663,#790,.T.);
#8111=EDGE_CURVE('',#6663,#6664,#3856,.T.);
#8112=EDGE_CURVE('',#6664,#6664,#791,.T.);
#8113=EDGE_CURVE('',#6665,#6665,#792,.T.);
#8114=EDGE_CURVE('',#6665,#6666,#3857,.T.);
#8115=EDGE_CURVE('',#6666,#6666,#793,.T.);
#8116=EDGE_CURVE('',#6667,#6667,#794,.T.);
#8117=EDGE_CURVE('',#6667,#6668,#3858,.T.);
#8118=EDGE_CURVE('',#6668,#6668,#795,.T.);
#8119=EDGE_CURVE('',#6669,#6669,#796,.T.);
#8120=EDGE_CURVE('',#6669,#6670,#3859,.T.);
#8121=EDGE_CURVE('',#6670,#6670,#797,.T.);
#8122=EDGE_CURVE('',#6671,#6671,#798,.T.);
#8123=EDGE_CURVE('',#6671,#6672,#3860,.T.);
#8124=EDGE_CURVE('',#6672,#6672,#799,.T.);
#8125=EDGE_CURVE('',#6673,#6673,#800,.T.);
#8126=EDGE_CURVE('',#6673,#6674,#3861,.T.);
#8127=EDGE_CURVE('',#6674,#6674,#801,.T.);
#8128=EDGE_CURVE('',#6675,#6675,#802,.T.);
#8129=EDGE_CURVE('',#6675,#6676,#3862,.T.);
#8130=EDGE_CURVE('',#6676,#6676,#803,.T.);
#8131=EDGE_CURVE('',#6677,#6677,#804,.T.);
#8132=EDGE_CURVE('',#6677,#6678,#3863,.T.);
#8133=EDGE_CURVE('',#6678,#6678,#805,.T.);
#8134=EDGE_CURVE('',#6679,#6679,#806,.T.);
#8135=EDGE_CURVE('',#6679,#6680,#3864,.T.);
#8136=EDGE_CURVE('',#6680,#6680,#807,.T.);
#8137=EDGE_CURVE('',#6681,#6681,#808,.T.);
#8138=EDGE_CURVE('',#6681,#6682,#3865,.T.);
#8139=EDGE_CURVE('',#6682,#6682,#809,.T.);
#8140=EDGE_CURVE('',#6683,#6683,#810,.T.);
#8141=EDGE_CURVE('',#6683,#6684,#3866,.T.);
#8142=EDGE_CURVE('',#6684,#6684,#811,.T.);
#8143=EDGE_CURVE('',#6685,#6685,#812,.T.);
#8144=EDGE_CURVE('',#6685,#6686,#3867,.T.);
#8145=EDGE_CURVE('',#6686,#6686,#813,.T.);
#8146=EDGE_CURVE('',#6687,#6687,#814,.T.);
#8147=EDGE_CURVE('',#6687,#6688,#3868,.T.);
#8148=EDGE_CURVE('',#6688,#6688,#815,.T.);
#8149=EDGE_CURVE('',#6689,#6689,#816,.T.);
#8150=EDGE_CURVE('',#6689,#6690,#3869,.T.);
#8151=EDGE_CURVE('',#6690,#6690,#817,.T.);
#8152=EDGE_CURVE('',#6691,#6691,#818,.T.);
#8153=EDGE_CURVE('',#6691,#6692,#3870,.T.);
#8154=EDGE_CURVE('',#6692,#6692,#819,.T.);
#10267=ORIENTED_EDGE('',*,*,#8017,.F.);
#10268=ORIENTED_EDGE('',*,*,#8018,.T.);
#10269=ORIENTED_EDGE('',*,*,#8019,.T.);
#10270=ORIENTED_EDGE('',*,*,#8018,.F.);
#10271=ORIENTED_EDGE('',*,*,#8020,.F.);
#10272=ORIENTED_EDGE('',*,*,#8021,.T.);
#10273=ORIENTED_EDGE('',*,*,#8022,.T.);
#10274=ORIENTED_EDGE('',*,*,#8021,.F.);
#10275=ORIENTED_EDGE('',*,*,#8023,.F.);
#10276=ORIENTED_EDGE('',*,*,#8024,.T.);
#10277=ORIENTED_EDGE('',*,*,#8025,.T.);
#10278=ORIENTED_EDGE('',*,*,#8024,.F.);
#10279=ORIENTED_EDGE('',*,*,#8026,.F.);
#10280=ORIENTED_EDGE('',*,*,#8027,.T.);
#10281=ORIENTED_EDGE('',*,*,#8028,.T.);
#10282=ORIENTED_EDGE('',*,*,#8027,.F.);
#10283=ORIENTED_EDGE('',*,*,#8029,.F.);
#10284=ORIENTED_EDGE('',*,*,#8030,.T.);
#10285=ORIENTED_EDGE('',*,*,#8031,.T.);
#10286=ORIENTED_EDGE('',*,*,#8030,.F.);
#10287=ORIENTED_EDGE('',*,*,#8032,.F.);
#10288=ORIENTED_EDGE('',*,*,#8033,.T.);
#10289=ORIENTED_EDGE('',*,*,#8034,.T.);
#10290=ORIENTED_EDGE('',*,*,#8033,.F.);
#10291=ORIENTED_EDGE('',*,*,#8035,.F.);
#10292=ORIENTED_EDGE('',*,*,#8036,.T.);
#10293=ORIENTED_EDGE('',*,*,#8037,.T.);
#10294=ORIENTED_EDGE('',*,*,#8036,.F.);
#10295=ORIENTED_EDGE('',*,*,#8038,.F.);
#10296=ORIENTED_EDGE('',*,*,#8039,.T.);
#10297=ORIENTED_EDGE('',*,*,#8040,.T.);
#10298=ORIENTED_EDGE('',*,*,#8039,.F.);
#10299=ORIENTED_EDGE('',*,*,#8041,.F.);
#10300=ORIENTED_EDGE('',*,*,#8042,.T.);
#10301=ORIENTED_EDGE('',*,*,#8043,.T.);
#10302=ORIENTED_EDGE('',*,*,#8042,.F.);
#10303=ORIENTED_EDGE('',*,*,#8044,.F.);
#10304=ORIENTED_EDGE('',*,*,#8045,.T.);
#10305=ORIENTED_EDGE('',*,*,#8046,.T.);
#10306=ORIENTED_EDGE('',*,*,#8045,.F.);
#10307=ORIENTED_EDGE('',*,*,#8047,.F.);
#10308=ORIENTED_EDGE('',*,*,#8048,.T.);
#10309=ORIENTED_EDGE('',*,*,#8049,.T.);
#10310=ORIENTED_EDGE('',*,*,#8048,.F.);
#10311=ORIENTED_EDGE('',*,*,#8050,.F.);
#10312=ORIENTED_EDGE('',*,*,#8051,.T.);
#10313=ORIENTED_EDGE('',*,*,#8052,.T.);
#10314=ORIENTED_EDGE('',*,*,#8051,.F.);
#10315=ORIENTED_EDGE('',*,*,#8053,.F.);
#10316=ORIENTED_EDGE('',*,*,#8054,.T.);
#10317=ORIENTED_EDGE('',*,*,#8055,.T.);
#10318=ORIENTED_EDGE('',*,*,#8054,.F.);
#10319=ORIENTED_EDGE('',*,*,#8056,.F.);
#10320=ORIENTED_EDGE('',*,*,#8057,.T.);
#10321=ORIENTED_EDGE('',*,*,#8058,.T.);
#10322=ORIENTED_EDGE('',*,*,#8057,.F.);
#10323=ORIENTED_EDGE('',*,*,#8059,.F.);
#10324=ORIENTED_EDGE('',*,*,#8060,.T.);
#10325=ORIENTED_EDGE('',*,*,#8061,.T.);
#10326=ORIENTED_EDGE('',*,*,#8060,.F.);
#10327=ORIENTED_EDGE('',*,*,#8062,.F.);
#10328=ORIENTED_EDGE('',*,*,#8063,.T.);
#10329=ORIENTED_EDGE('',*,*,#8064,.T.);
#10330=ORIENTED_EDGE('',*,*,#8063,.F.);
#10331=ORIENTED_EDGE('',*,*,#8065,.F.);
#10332=ORIENTED_EDGE('',*,*,#8066,.T.);
#10333=ORIENTED_EDGE('',*,*,#8067,.T.);
#10334=ORIENTED_EDGE('',*,*,#8066,.F.);
#10335=ORIENTED_EDGE('',*,*,#8068,.F.);
#10336=ORIENTED_EDGE('',*,*,#8069,.T.);
#10337=ORIENTED_EDGE('',*,*,#8070,.T.);
#10338=ORIENTED_EDGE('',*,*,#8069,.F.);
#10339=ORIENTED_EDGE('',*,*,#8071,.F.);
#10340=ORIENTED_EDGE('',*,*,#8072,.F.);
#10341=ORIENTED_EDGE('',*,*,#8073,.T.);
#10342=ORIENTED_EDGE('',*,*,#8074,.T.);
#10343=ORIENTED_EDGE('',*,*,#8075,.F.);
#10344=ORIENTED_EDGE('',*,*,#8076,.F.);
#10345=ORIENTED_EDGE('',*,*,#8077,.T.);
#10346=ORIENTED_EDGE('',*,*,#8072,.T.);
#10347=ORIENTED_EDGE('',*,*,#8078,.F.);
#10348=ORIENTED_EDGE('',*,*,#8079,.F.);
#10349=ORIENTED_EDGE('',*,*,#8080,.T.);
#10350=ORIENTED_EDGE('',*,*,#8076,.T.);
#10351=ORIENTED_EDGE('',*,*,#8081,.F.);
#10352=ORIENTED_EDGE('',*,*,#8074,.F.);
#10353=ORIENTED_EDGE('',*,*,#8082,.T.);
#10354=ORIENTED_EDGE('',*,*,#8079,.T.);
#10355=ORIENTED_EDGE('',*,*,#8073,.F.);
#10356=ORIENTED_EDGE('',*,*,#8077,.F.);
#10357=ORIENTED_EDGE('',*,*,#8080,.F.);
#10358=ORIENTED_EDGE('',*,*,#8082,.F.);
#10359=ORIENTED_EDGE('',*,*,#8017,.T.);
#10360=ORIENTED_EDGE('',*,*,#8020,.T.);
#10361=ORIENTED_EDGE('',*,*,#8023,.T.);
#10362=ORIENTED_EDGE('',*,*,#8026,.T.);
#10363=ORIENTED_EDGE('',*,*,#8029,.T.);
#10364=ORIENTED_EDGE('',*,*,#8032,.T.);
#10365=ORIENTED_EDGE('',*,*,#8035,.T.);
#10366=ORIENTED_EDGE('',*,*,#8038,.T.);
#10367=ORIENTED_EDGE('',*,*,#8041,.T.);
#10368=ORIENTED_EDGE('',*,*,#8044,.T.);
#10369=ORIENTED_EDGE('',*,*,#8047,.T.);
#10370=ORIENTED_EDGE('',*,*,#8050,.T.);
#10371=ORIENTED_EDGE('',*,*,#8053,.T.);
#10372=ORIENTED_EDGE('',*,*,#8056,.T.);
#10373=ORIENTED_EDGE('',*,*,#8059,.T.);
#10374=ORIENTED_EDGE('',*,*,#8062,.T.);
#10375=ORIENTED_EDGE('',*,*,#8065,.T.);
#10376=ORIENTED_EDGE('',*,*,#8068,.T.);
#10377=ORIENTED_EDGE('',*,*,#8071,.T.);
#10378=ORIENTED_EDGE('',*,*,#8081,.T.);
#10379=ORIENTED_EDGE('',*,*,#8078,.T.);
#10380=ORIENTED_EDGE('',*,*,#8075,.T.);
#10381=ORIENTED_EDGE('',*,*,#8019,.F.);
#10382=ORIENTED_EDGE('',*,*,#8022,.F.);
#10383=ORIENTED_EDGE('',*,*,#8025,.F.);
#10384=ORIENTED_EDGE('',*,*,#8028,.F.);
#10385=ORIENTED_EDGE('',*,*,#8031,.F.);
#10386=ORIENTED_EDGE('',*,*,#8034,.F.);
#10387=ORIENTED_EDGE('',*,*,#8037,.F.);
#10388=ORIENTED_EDGE('',*,*,#8040,.F.);
#10389=ORIENTED_EDGE('',*,*,#8043,.F.);
#10390=ORIENTED_EDGE('',*,*,#8046,.F.);
#10391=ORIENTED_EDGE('',*,*,#8049,.F.);
#10392=ORIENTED_EDGE('',*,*,#8052,.F.);
#10393=ORIENTED_EDGE('',*,*,#8055,.F.);
#10394=ORIENTED_EDGE('',*,*,#8058,.F.);
#10395=ORIENTED_EDGE('',*,*,#8061,.F.);
#10396=ORIENTED_EDGE('',*,*,#8064,.F.);
#10397=ORIENTED_EDGE('',*,*,#8067,.F.);
#10398=ORIENTED_EDGE('',*,*,#8070,.F.);
#10399=ORIENTED_EDGE('',*,*,#8083,.T.);
#10400=ORIENTED_EDGE('',*,*,#8084,.T.);
#10401=ORIENTED_EDGE('',*,*,#8085,.F.);
#10402=ORIENTED_EDGE('',*,*,#8084,.F.);
#10403=ORIENTED_EDGE('',*,*,#8086,.T.);
#10404=ORIENTED_EDGE('',*,*,#8087,.T.);
#10405=ORIENTED_EDGE('',*,*,#8088,.F.);
#10406=ORIENTED_EDGE('',*,*,#8087,.F.);
#10407=ORIENTED_EDGE('',*,*,#8085,.T.);
#10408=ORIENTED_EDGE('',*,*,#8086,.F.);
#10409=ORIENTED_EDGE('',*,*,#8083,.F.);
#10410=ORIENTED_EDGE('',*,*,#8088,.T.);
#10411=ORIENTED_EDGE('',*,*,#8089,.T.);
#10412=ORIENTED_EDGE('',*,*,#8090,.T.);
#10413=ORIENTED_EDGE('',*,*,#8091,.F.);
#10414=ORIENTED_EDGE('',*,*,#8090,.F.);
#10415=ORIENTED_EDGE('',*,*,#8092,.T.);
#10416=ORIENTED_EDGE('',*,*,#8093,.T.);
#10417=ORIENTED_EDGE('',*,*,#8094,.F.);
#10418=ORIENTED_EDGE('',*,*,#8093,.F.);
#10419=ORIENTED_EDGE('',*,*,#8091,.T.);
#10420=ORIENTED_EDGE('',*,*,#8092,.F.);
#10421=ORIENTED_EDGE('',*,*,#8089,.F.);
#10422=ORIENTED_EDGE('',*,*,#8094,.T.);
#10423=ORIENTED_EDGE('',*,*,#8095,.F.);
#10424=ORIENTED_EDGE('',*,*,#8096,.T.);
#10425=ORIENTED_EDGE('',*,*,#8097,.T.);
#10426=ORIENTED_EDGE('',*,*,#8096,.F.);
#10427=ORIENTED_EDGE('',*,*,#8098,.F.);
#10428=ORIENTED_EDGE('',*,*,#8099,.T.);
#10429=ORIENTED_EDGE('',*,*,#8100,.T.);
#10430=ORIENTED_EDGE('',*,*,#8099,.F.);
#10431=ORIENTED_EDGE('',*,*,#8101,.F.);
#10432=ORIENTED_EDGE('',*,*,#8102,.T.);
#10433=ORIENTED_EDGE('',*,*,#8103,.T.);
#10434=ORIENTED_EDGE('',*,*,#8102,.F.);
#10435=ORIENTED_EDGE('',*,*,#8104,.F.);
#10436=ORIENTED_EDGE('',*,*,#8105,.T.);
#10437=ORIENTED_EDGE('',*,*,#8106,.T.);
#10438=ORIENTED_EDGE('',*,*,#8105,.F.);
#10439=ORIENTED_EDGE('',*,*,#8107,.F.);
#10440=ORIENTED_EDGE('',*,*,#8108,.T.);
#10441=ORIENTED_EDGE('',*,*,#8109,.T.);
#10442=ORIENTED_EDGE('',*,*,#8108,.F.);
#10443=ORIENTED_EDGE('',*,*,#8110,.F.);
#10444=ORIENTED_EDGE('',*,*,#8111,.T.);
#10445=ORIENTED_EDGE('',*,*,#8112,.T.);
#10446=ORIENTED_EDGE('',*,*,#8111,.F.);
#10447=ORIENTED_EDGE('',*,*,#8113,.F.);
#10448=ORIENTED_EDGE('',*,*,#8114,.T.);
#10449=ORIENTED_EDGE('',*,*,#8115,.T.);
#10450=ORIENTED_EDGE('',*,*,#8114,.F.);
#10451=ORIENTED_EDGE('',*,*,#8116,.F.);
#10452=ORIENTED_EDGE('',*,*,#8117,.T.);
#10453=ORIENTED_EDGE('',*,*,#8118,.T.);
#10454=ORIENTED_EDGE('',*,*,#8117,.F.);
#10455=ORIENTED_EDGE('',*,*,#8119,.F.);
#10456=ORIENTED_EDGE('',*,*,#8120,.T.);
#10457=ORIENTED_EDGE('',*,*,#8121,.T.);
#10458=ORIENTED_EDGE('',*,*,#8120,.F.);
#10459=ORIENTED_EDGE('',*,*,#8122,.F.);
#10460=ORIENTED_EDGE('',*,*,#8123,.T.);
#10461=ORIENTED_EDGE('',*,*,#8124,.T.);
#10462=ORIENTED_EDGE('',*,*,#8123,.F.);
#10463=ORIENTED_EDGE('',*,*,#8125,.F.);
#10464=ORIENTED_EDGE('',*,*,#8126,.T.);
#10465=ORIENTED_EDGE('',*,*,#8127,.T.);
#10466=ORIENTED_EDGE('',*,*,#8126,.F.);
#10467=ORIENTED_EDGE('',*,*,#8128,.F.);
#10468=ORIENTED_EDGE('',*,*,#8129,.T.);
#10469=ORIENTED_EDGE('',*,*,#8130,.T.);
#10470=ORIENTED_EDGE('',*,*,#8129,.F.);
#10471=ORIENTED_EDGE('',*,*,#8131,.F.);
#10472=ORIENTED_EDGE('',*,*,#8132,.T.);
#10473=ORIENTED_EDGE('',*,*,#8133,.T.);
#10474=ORIENTED_EDGE('',*,*,#8132,.F.);
#10475=ORIENTED_EDGE('',*,*,#8134,.F.);
#10476=ORIENTED_EDGE('',*,*,#8135,.T.);
#10477=ORIENTED_EDGE('',*,*,#8136,.T.);
#10478=ORIENTED_EDGE('',*,*,#8135,.F.);
#10479=ORIENTED_EDGE('',*,*,#8136,.F.);
#10480=ORIENTED_EDGE('',*,*,#8095,.T.);
#10481=ORIENTED_EDGE('',*,*,#8098,.T.);
#10482=ORIENTED_EDGE('',*,*,#8101,.T.);
#10483=ORIENTED_EDGE('',*,*,#8104,.T.);
#10484=ORIENTED_EDGE('',*,*,#8107,.T.);
#10485=ORIENTED_EDGE('',*,*,#8110,.T.);
#10486=ORIENTED_EDGE('',*,*,#8113,.T.);
#10487=ORIENTED_EDGE('',*,*,#8116,.T.);
#10488=ORIENTED_EDGE('',*,*,#8119,.T.);
#10489=ORIENTED_EDGE('',*,*,#8122,.T.);
#10490=ORIENTED_EDGE('',*,*,#8125,.T.);
#10491=ORIENTED_EDGE('',*,*,#8128,.T.);
#10492=ORIENTED_EDGE('',*,*,#8131,.T.);
#10493=ORIENTED_EDGE('',*,*,#8134,.T.);
#10494=ORIENTED_EDGE('',*,*,#8097,.F.);
#10495=ORIENTED_EDGE('',*,*,#8100,.F.);
#10496=ORIENTED_EDGE('',*,*,#8103,.F.);
#10497=ORIENTED_EDGE('',*,*,#8106,.F.);
#10498=ORIENTED_EDGE('',*,*,#8109,.F.);
#10499=ORIENTED_EDGE('',*,*,#8112,.F.);
#10500=ORIENTED_EDGE('',*,*,#8115,.F.);
#10501=ORIENTED_EDGE('',*,*,#8118,.F.);
#10502=ORIENTED_EDGE('',*,*,#8121,.F.);
#10503=ORIENTED_EDGE('',*,*,#8124,.F.);
#10504=ORIENTED_EDGE('',*,*,#8127,.F.);
#10505=ORIENTED_EDGE('',*,*,#8130,.F.);
#10506=ORIENTED_EDGE('',*,*,#8133,.F.);
#10507=ORIENTED_EDGE('',*,*,#8137,.F.);
#10508=ORIENTED_EDGE('',*,*,#8138,.T.);
#10509=ORIENTED_EDGE('',*,*,#8139,.T.);
#10510=ORIENTED_EDGE('',*,*,#8138,.F.);
#10511=ORIENTED_EDGE('',*,*,#8140,.F.);
#10512=ORIENTED_EDGE('',*,*,#8141,.T.);
#10513=ORIENTED_EDGE('',*,*,#8142,.T.);
#10514=ORIENTED_EDGE('',*,*,#8141,.F.);
#10515=ORIENTED_EDGE('',*,*,#8143,.F.);
#10516=ORIENTED_EDGE('',*,*,#8144,.T.);
#10517=ORIENTED_EDGE('',*,*,#8145,.T.);
#10518=ORIENTED_EDGE('',*,*,#8144,.F.);
#10519=ORIENTED_EDGE('',*,*,#8146,.F.);
#10520=ORIENTED_EDGE('',*,*,#8147,.T.);
#10521=ORIENTED_EDGE('',*,*,#8148,.T.);
#10522=ORIENTED_EDGE('',*,*,#8147,.F.);
#10523=ORIENTED_EDGE('',*,*,#8149,.F.);
#10524=ORIENTED_EDGE('',*,*,#8150,.T.);
#10525=ORIENTED_EDGE('',*,*,#8151,.T.);
#10526=ORIENTED_EDGE('',*,*,#8150,.F.);
#10527=ORIENTED_EDGE('',*,*,#8152,.F.);
#10528=ORIENTED_EDGE('',*,*,#8153,.T.);
#10529=ORIENTED_EDGE('',*,*,#8154,.T.);
#10530=ORIENTED_EDGE('',*,*,#8153,.F.);
#10531=ORIENTED_EDGE('',*,*,#8154,.F.);
#10532=ORIENTED_EDGE('',*,*,#8137,.T.);
#10533=ORIENTED_EDGE('',*,*,#8140,.T.);
#10534=ORIENTED_EDGE('',*,*,#8143,.T.);
#10535=ORIENTED_EDGE('',*,*,#8146,.T.);
#10536=ORIENTED_EDGE('',*,*,#8149,.T.);
#10537=ORIENTED_EDGE('',*,*,#8152,.T.);
#10538=ORIENTED_EDGE('',*,*,#8139,.F.);
#10539=ORIENTED_EDGE('',*,*,#8142,.F.);
#10540=ORIENTED_EDGE('',*,*,#8145,.F.);
#10541=ORIENTED_EDGE('',*,*,#8148,.F.);
#10542=ORIENTED_EDGE('',*,*,#8151,.F.);
#14107=PLANE('',#15954);
#14108=PLANE('',#15955);
#14109=PLANE('',#15956);
#14110=PLANE('',#15957);
#14111=PLANE('',#15958);
#14112=PLANE('',#15959);
#14113=PLANE('',#15966);
#14114=PLANE('',#15967);
#14115=PLANE('',#15974);
#14116=PLANE('',#15975);
#14117=PLANE('',#16018);
#14118=PLANE('',#16019);
#14119=PLANE('',#16038);
#14120=PLANE('',#16039);
#14722=ADVANCED_FACE('',(#1754),#1099,.F.);
#14723=ADVANCED_FACE('',(#1755),#1100,.F.);
#14724=ADVANCED_FACE('',(#1756),#1101,.F.);
#14725=ADVANCED_FACE('',(#1757),#1102,.F.);
#14726=ADVANCED_FACE('',(#1758),#1103,.F.);
#14727=ADVANCED_FACE('',(#1759),#1104,.F.);
#14728=ADVANCED_FACE('',(#1760),#1105,.F.);
#14729=ADVANCED_FACE('',(#1761),#1106,.F.);
#14730=ADVANCED_FACE('',(#1762),#1107,.F.);
#14731=ADVANCED_FACE('',(#1763),#1108,.F.);
#14732=ADVANCED_FACE('',(#1764),#1109,.F.);
#14733=ADVANCED_FACE('',(#1765),#1110,.F.);
#14734=ADVANCED_FACE('',(#1766),#1111,.F.);
#14735=ADVANCED_FACE('',(#1767),#1112,.F.);
#14736=ADVANCED_FACE('',(#1768),#1113,.F.);
#14737=ADVANCED_FACE('',(#1769),#1114,.F.);
#14738=ADVANCED_FACE('',(#1770),#1115,.F.);
#14739=ADVANCED_FACE('',(#1771),#1116,.F.);
#14740=ADVANCED_FACE('',(#1772),#14107,.T.);
#14741=ADVANCED_FACE('',(#1773),#14108,.T.);
#14742=ADVANCED_FACE('',(#1774),#14109,.T.);
#14743=ADVANCED_FACE('',(#1775),#14110,.T.);
#14744=ADVANCED_FACE('',(#1776,#1503,#1504,#1505,#1506,#1507,#1508,#1509,
#1510,#1511,#1512,#1513,#1514,#1515,#1516,#1517,#1518,#1519,#1520),#14111,
 .T.);
#14745=ADVANCED_FACE('',(#1777,#1521,#1522,#1523,#1524,#1525,#1526,#1527,
#1528,#1529,#1530,#1531,#1532,#1533,#1534,#1535,#1536,#1537,#1538),#14112,
 .F.);
#14746=ADVANCED_FACE('',(#1778),#1117,.T.);
#14747=ADVANCED_FACE('',(#1779),#1118,.F.);
#14748=ADVANCED_FACE('',(#1780,#1539),#14113,.T.);
#14749=ADVANCED_FACE('',(#1781,#1540),#14114,.F.);
#14750=ADVANCED_FACE('',(#1782),#1119,.T.);
#14751=ADVANCED_FACE('',(#1783),#1120,.F.);
#14752=ADVANCED_FACE('',(#1784,#1541),#14115,.T.);
#14753=ADVANCED_FACE('',(#1785,#1542),#14116,.F.);
#14754=ADVANCED_FACE('',(#1786),#1121,.F.);
#14755=ADVANCED_FACE('',(#1787),#1122,.F.);
#14756=ADVANCED_FACE('',(#1788),#1123,.F.);
#14757=ADVANCED_FACE('',(#1789),#1124,.F.);
#14758=ADVANCED_FACE('',(#1790),#1125,.F.);
#14759=ADVANCED_FACE('',(#1791),#1126,.F.);
#14760=ADVANCED_FACE('',(#1792),#1127,.F.);
#14761=ADVANCED_FACE('',(#1793),#1128,.F.);
#14762=ADVANCED_FACE('',(#1794),#1129,.F.);
#14763=ADVANCED_FACE('',(#1795),#1130,.F.);
#14764=ADVANCED_FACE('',(#1796),#1131,.F.);
#14765=ADVANCED_FACE('',(#1797),#1132,.F.);
#14766=ADVANCED_FACE('',(#1798),#1133,.F.);
#14767=ADVANCED_FACE('',(#1799),#1134,.T.);
#14768=ADVANCED_FACE('',(#1800,#1543,#1544,#1545,#1546,#1547,#1548,#1549,
#1550,#1551,#1552,#1553,#1554,#1555),#14117,.F.);
#14769=ADVANCED_FACE('',(#1801,#1556,#1557,#1558,#1559,#1560,#1561,#1562,
#1563,#1564,#1565,#1566,#1567,#1568),#14118,.T.);
#14770=ADVANCED_FACE('',(#1802),#1135,.F.);
#14771=ADVANCED_FACE('',(#1803),#1136,.F.);
#14772=ADVANCED_FACE('',(#1804),#1137,.F.);
#14773=ADVANCED_FACE('',(#1805),#1138,.F.);
#14774=ADVANCED_FACE('',(#1806),#1139,.F.);
#14775=ADVANCED_FACE('',(#1807),#1140,.T.);
#14776=ADVANCED_FACE('',(#1808,#1569,#1570,#1571,#1572,#1573),#14119,.F.);
#14777=ADVANCED_FACE('',(#1809,#1574,#1575,#1576,#1577,#1578),#14120,.T.);
#15548=CLOSED_SHELL('',(#14722,#14723,#14724,#14725,#14726,#14727,#14728,
#14729,#14730,#14731,#14732,#14733,#14734,#14735,#14736,#14737,#14738,#14739,
#14740,#14741,#14742,#14743,#14744,#14745));
#15549=CLOSED_SHELL('',(#14746,#14747,#14748,#14749));
#15550=CLOSED_SHELL('',(#14750,#14751,#14752,#14753));
#15551=CLOSED_SHELL('',(#14754,#14755,#14756,#14757,#14758,#14759,#14760,
#14761,#14762,#14763,#14764,#14765,#14766,#14767,#14768,#14769));
#15552=CLOSED_SHELL('',(#14770,#14771,#14772,#14773,#14774,#14775,#14776,
#14777));
#15899=AXIS2_PLACEMENT_3D('',#21689,#17533,#17534);
#15900=AXIS2_PLACEMENT_3D('',#21690,#17535,#17536);
#15901=AXIS2_PLACEMENT_3D('',#21692,#17537,#17538);
#15902=AXIS2_PLACEMENT_3D('',#21695,#17540,#17541);
#15903=AXIS2_PLACEMENT_3D('',#21696,#17542,#17543);
#15904=AXIS2_PLACEMENT_3D('',#21698,#17544,#17545);
#15905=AXIS2_PLACEMENT_3D('',#21701,#17547,#17548);
#15906=AXIS2_PLACEMENT_3D('',#21702,#17549,#17550);
#15907=AXIS2_PLACEMENT_3D('',#21704,#17551,#17552);
#15908=AXIS2_PLACEMENT_3D('',#21707,#17554,#17555);
#15909=AXIS2_PLACEMENT_3D('',#21708,#17556,#17557);
#15910=AXIS2_PLACEMENT_3D('',#21710,#17558,#17559);
#15911=AXIS2_PLACEMENT_3D('',#21713,#17561,#17562);
#15912=AXIS2_PLACEMENT_3D('',#21714,#17563,#17564);
#15913=AXIS2_PLACEMENT_3D('',#21716,#17565,#17566);
#15914=AXIS2_PLACEMENT_3D('',#21719,#17568,#17569);
#15915=AXIS2_PLACEMENT_3D('',#21720,#17570,#17571);
#15916=AXIS2_PLACEMENT_3D('',#21722,#17572,#17573);
#15917=AXIS2_PLACEMENT_3D('',#21725,#17575,#17576);
#15918=AXIS2_PLACEMENT_3D('',#21726,#17577,#17578);
#15919=AXIS2_PLACEMENT_3D('',#21728,#17579,#17580);
#15920=AXIS2_PLACEMENT_3D('',#21731,#17582,#17583);
#15921=AXIS2_PLACEMENT_3D('',#21732,#17584,#17585);
#15922=AXIS2_PLACEMENT_3D('',#21734,#17586,#17587);
#15923=AXIS2_PLACEMENT_3D('',#21737,#17589,#17590);
#15924=AXIS2_PLACEMENT_3D('',#21738,#17591,#17592);
#15925=AXIS2_PLACEMENT_3D('',#21740,#17593,#17594);
#15926=AXIS2_PLACEMENT_3D('',#21743,#17596,#17597);
#15927=AXIS2_PLACEMENT_3D('',#21744,#17598,#17599);
#15928=AXIS2_PLACEMENT_3D('',#21746,#17600,#17601);
#15929=AXIS2_PLACEMENT_3D('',#21749,#17603,#17604);
#15930=AXIS2_PLACEMENT_3D('',#21750,#17605,#17606);
#15931=AXIS2_PLACEMENT_3D('',#21752,#17607,#17608);
#15932=AXIS2_PLACEMENT_3D('',#21755,#17610,#17611);
#15933=AXIS2_PLACEMENT_3D('',#21756,#17612,#17613);
#15934=AXIS2_PLACEMENT_3D('',#21758,#17614,#17615);
#15935=AXIS2_PLACEMENT_3D('',#21761,#17617,#17618);
#15936=AXIS2_PLACEMENT_3D('',#21762,#17619,#17620);
#15937=AXIS2_PLACEMENT_3D('',#21764,#17621,#17622);
#15938=AXIS2_PLACEMENT_3D('',#21767,#17624,#17625);
#15939=AXIS2_PLACEMENT_3D('',#21768,#17626,#17627);
#15940=AXIS2_PLACEMENT_3D('',#21770,#17628,#17629);
#15941=AXIS2_PLACEMENT_3D('',#21773,#17631,#17632);
#15942=AXIS2_PLACEMENT_3D('',#21774,#17633,#17634);
#15943=AXIS2_PLACEMENT_3D('',#21776,#17635,#17636);
#15944=AXIS2_PLACEMENT_3D('',#21779,#17638,#17639);
#15945=AXIS2_PLACEMENT_3D('',#21780,#17640,#17641);
#15946=AXIS2_PLACEMENT_3D('',#21782,#17642,#17643);
#15947=AXIS2_PLACEMENT_3D('',#21785,#17645,#17646);
#15948=AXIS2_PLACEMENT_3D('',#21786,#17647,#17648);
#15949=AXIS2_PLACEMENT_3D('',#21788,#17649,#17650);
#15950=AXIS2_PLACEMENT_3D('',#21791,#17652,#17653);
#15951=AXIS2_PLACEMENT_3D('',#21792,#17654,#17655);
#15952=AXIS2_PLACEMENT_3D('',#21794,#17656,#17657);
#15953=AXIS2_PLACEMENT_3D('',#21797,#17659,#17660);
#15954=AXIS2_PLACEMENT_3D('',#21798,#17661,#17662);
#15955=AXIS2_PLACEMENT_3D('',#21807,#17667,#17668);
#15956=AXIS2_PLACEMENT_3D('',#21813,#17672,#17673);
#15957=AXIS2_PLACEMENT_3D('',#21819,#17677,#17678);
#15958=AXIS2_PLACEMENT_3D('',#21822,#17681,#17682);
#15959=AXIS2_PLACEMENT_3D('',#21823,#17683,#17684);
#15960=AXIS2_PLACEMENT_3D('',#21824,#17685,#17686);
#15961=AXIS2_PLACEMENT_3D('',#21826,#17687,#17688);
#15962=AXIS2_PLACEMENT_3D('',#21829,#17690,#17691);
#15963=AXIS2_PLACEMENT_3D('',#21830,#17692,#17693);
#15964=AXIS2_PLACEMENT_3D('',#21832,#17694,#17695);
#15965=AXIS2_PLACEMENT_3D('',#21835,#17697,#17698);
#15966=AXIS2_PLACEMENT_3D('',#21836,#17699,#17700);
#15967=AXIS2_PLACEMENT_3D('',#21837,#17701,#17702);
#15968=AXIS2_PLACEMENT_3D('',#21838,#17703,#17704);
#15969=AXIS2_PLACEMENT_3D('',#21840,#17705,#17706);
#15970=AXIS2_PLACEMENT_3D('',#21843,#17708,#17709);
#15971=AXIS2_PLACEMENT_3D('',#21844,#17710,#17711);
#15972=AXIS2_PLACEMENT_3D('',#21846,#17712,#17713);
#15973=AXIS2_PLACEMENT_3D('',#21849,#17715,#17716);
#15974=AXIS2_PLACEMENT_3D('',#21850,#17717,#17718);
#15975=AXIS2_PLACEMENT_3D('',#21851,#17719,#17720);
#15976=AXIS2_PLACEMENT_3D('',#21852,#17721,#17722);
#15977=AXIS2_PLACEMENT_3D('',#21854,#17723,#17724);
#15978=AXIS2_PLACEMENT_3D('',#21857,#17726,#17727);
#15979=AXIS2_PLACEMENT_3D('',#21858,#17728,#17729);
#15980=AXIS2_PLACEMENT_3D('',#21860,#17730,#17731);
#15981=AXIS2_PLACEMENT_3D('',#21863,#17733,#17734);
#15982=AXIS2_PLACEMENT_3D('',#21864,#17735,#17736);
#15983=AXIS2_PLACEMENT_3D('',#21866,#17737,#17738);
#15984=AXIS2_PLACEMENT_3D('',#21869,#17740,#17741);
#15985=AXIS2_PLACEMENT_3D('',#21870,#17742,#17743);
#15986=AXIS2_PLACEMENT_3D('',#21872,#17744,#17745);
#15987=AXIS2_PLACEMENT_3D('',#21875,#17747,#17748);
#15988=AXIS2_PLACEMENT_3D('',#21876,#17749,#17750);
#15989=AXIS2_PLACEMENT_3D('',#21878,#17751,#17752);
#15990=AXIS2_PLACEMENT_3D('',#21881,#17754,#17755);
#15991=AXIS2_PLACEMENT_3D('',#21882,#17756,#17757);
#15992=AXIS2_PLACEMENT_3D('',#21884,#17758,#17759);
#15993=AXIS2_PLACEMENT_3D('',#21887,#17761,#17762);
#15994=AXIS2_PLACEMENT_3D('',#21888,#17763,#17764);
#15995=AXIS2_PLACEMENT_3D('',#21890,#17765,#17766);
#15996=AXIS2_PLACEMENT_3D('',#21893,#17768,#17769);
#15997=AXIS2_PLACEMENT_3D('',#21894,#17770,#17771);
#15998=AXIS2_PLACEMENT_3D('',#21896,#17772,#17773);
#15999=AXIS2_PLACEMENT_3D('',#21899,#17775,#17776);
#16000=AXIS2_PLACEMENT_3D('',#21900,#17777,#17778);
#16001=AXIS2_PLACEMENT_3D('',#21902,#17779,#17780);
#16002=AXIS2_PLACEMENT_3D('',#21905,#17782,#17783);
#16003=AXIS2_PLACEMENT_3D('',#21906,#17784,#17785);
#16004=AXIS2_PLACEMENT_3D('',#21908,#17786,#17787);
#16005=AXIS2_PLACEMENT_3D('',#21911,#17789,#17790);
#16006=AXIS2_PLACEMENT_3D('',#21912,#17791,#17792);
#16007=AXIS2_PLACEMENT_3D('',#21914,#17793,#17794);
#16008=AXIS2_PLACEMENT_3D('',#21917,#17796,#17797);
#16009=AXIS2_PLACEMENT_3D('',#21918,#17798,#17799);
#16010=AXIS2_PLACEMENT_3D('',#21920,#17800,#17801);
#16011=AXIS2_PLACEMENT_3D('',#21923,#17803,#17804);
#16012=AXIS2_PLACEMENT_3D('',#21924,#17805,#17806);
#16013=AXIS2_PLACEMENT_3D('',#21926,#17807,#17808);
#16014=AXIS2_PLACEMENT_3D('',#21929,#17810,#17811);
#16015=AXIS2_PLACEMENT_3D('',#21930,#17812,#17813);
#16016=AXIS2_PLACEMENT_3D('',#21932,#17814,#17815);
#16017=AXIS2_PLACEMENT_3D('',#21935,#17817,#17818);
#16018=AXIS2_PLACEMENT_3D('',#21936,#17819,#17820);
#16019=AXIS2_PLACEMENT_3D('',#21937,#17821,#17822);
#16020=AXIS2_PLACEMENT_3D('',#21938,#17823,#17824);
#16021=AXIS2_PLACEMENT_3D('',#21940,#17825,#17826);
#16022=AXIS2_PLACEMENT_3D('',#21943,#17828,#17829);
#16023=AXIS2_PLACEMENT_3D('',#21944,#17830,#17831);
#16024=AXIS2_PLACEMENT_3D('',#21946,#17832,#17833);
#16025=AXIS2_PLACEMENT_3D('',#21949,#17835,#17836);
#16026=AXIS2_PLACEMENT_3D('',#21950,#17837,#17838);
#16027=AXIS2_PLACEMENT_3D('',#21952,#17839,#17840);
#16028=AXIS2_PLACEMENT_3D('',#21955,#17842,#17843);
#16029=AXIS2_PLACEMENT_3D('',#21956,#17844,#17845);
#16030=AXIS2_PLACEMENT_3D('',#21958,#17846,#17847);
#16031=AXIS2_PLACEMENT_3D('',#21961,#17849,#17850);
#16032=AXIS2_PLACEMENT_3D('',#21962,#17851,#17852);
#16033=AXIS2_PLACEMENT_3D('',#21964,#17853,#17854);
#16034=AXIS2_PLACEMENT_3D('',#21967,#17856,#17857);
#16035=AXIS2_PLACEMENT_3D('',#21968,#17858,#17859);
#16036=AXIS2_PLACEMENT_3D('',#21970,#17860,#17861);
#16037=AXIS2_PLACEMENT_3D('',#21973,#17863,#17864);
#16038=AXIS2_PLACEMENT_3D('',#21974,#17865,#17866);
#16039=AXIS2_PLACEMENT_3D('',#21975,#17867,#17868);
#17533=DIRECTION('axis',(0.,0.,1.));
#17534=DIRECTION('refdir',(1.,0.,0.));
#17535=DIRECTION('center_axis',(9.93056848476794E-32,1.,-3.33066907387547E-16));
#17536=DIRECTION('ref_axis',(7.13571935167128E-47,3.33066907387547E-16,
1.));
#17537=DIRECTION('center_axis',(9.93056848476794E-32,1.,-3.33066907387547E-16));
#17538=DIRECTION('ref_axis',(7.13571935167128E-47,3.33066907387547E-16,
1.));
#17539=DIRECTION('',(9.93056848476794E-32,1.,-3.33066907387547E-16));
#17540=DIRECTION('center_axis',(9.93056848476794E-32,1.,-3.33066907387547E-16));
#17541=DIRECTION('ref_axis',(6.61508746764379E-47,3.33066907387547E-16,
1.));
#17542=DIRECTION('center_axis',(9.93056848476794E-32,1.,-3.33066907387547E-16));
#17543=DIRECTION('ref_axis',(7.13571935167128E-47,3.33066907387547E-16,
1.));
#17544=DIRECTION('center_axis',(9.93056848476794E-32,1.,-3.33066907387547E-16));
#17545=DIRECTION('ref_axis',(7.13571935167128E-47,3.33066907387547E-16,
1.));
#17546=DIRECTION('',(9.93056848476794E-32,1.,-3.33066907387547E-16));
#17547=DIRECTION('center_axis',(9.93056848476794E-32,1.,-3.33066907387547E-16));
#17548=DIRECTION('ref_axis',(6.61508746764379E-47,3.33066907387547E-16,
1.));
#17549=DIRECTION('center_axis',(9.93056848476794E-32,1.,-3.33066907387547E-16));
#17550=DIRECTION('ref_axis',(7.13571935167129E-47,3.33066907387547E-16,
1.));
#17551=DIRECTION('center_axis',(9.93056848476794E-32,1.,-3.33066907387547E-16));
#17552=DIRECTION('ref_axis',(7.13571935167129E-47,3.33066907387547E-16,
1.));
#17553=DIRECTION('',(9.93056848476794E-32,1.,-3.33066907387547E-16));
#17554=DIRECTION('center_axis',(9.93056848476794E-32,1.,-3.33066907387547E-16));
#17555=DIRECTION('ref_axis',(6.61508746764379E-47,3.33066907387547E-16,
1.));
#17556=DIRECTION('center_axis',(9.93056848476794E-32,1.,-3.33066907387547E-16));
#17557=DIRECTION('ref_axis',(7.13571935167129E-47,3.33066907387547E-16,
1.));
#17558=DIRECTION('center_axis',(9.93056848476794E-32,1.,-3.33066907387547E-16));
#17559=DIRECTION('ref_axis',(7.13571935167129E-47,3.33066907387547E-16,
1.));
#17560=DIRECTION('',(9.93056848476794E-32,1.,-3.33066907387547E-16));
#17561=DIRECTION('center_axis',(9.93056848476794E-32,1.,-3.33066907387547E-16));
#17562=DIRECTION('ref_axis',(6.61508746764379E-47,3.33066907387547E-16,
1.));
#17563=DIRECTION('center_axis',(9.93056848476794E-32,1.,-3.33066907387547E-16));
#17564=DIRECTION('ref_axis',(7.13571935167128E-47,3.33066907387547E-16,
1.));
#17565=DIRECTION('center_axis',(9.93056848476794E-32,1.,-3.33066907387547E-16));
#17566=DIRECTION('ref_axis',(7.13571935167128E-47,3.33066907387547E-16,
1.));
#17567=DIRECTION('',(9.93056848476794E-32,1.,-3.33066907387547E-16));
#17568=DIRECTION('center_axis',(9.93056848476794E-32,1.,-3.33066907387547E-16));
#17569=DIRECTION('ref_axis',(6.61508746764379E-47,3.33066907387547E-16,
1.));
#17570=DIRECTION('center_axis',(9.93056848476794E-32,1.,-3.33066907387547E-16));
#17571=DIRECTION('ref_axis',(7.13571935167128E-47,3.33066907387547E-16,
1.));
#17572=DIRECTION('center_axis',(9.93056848476794E-32,1.,-3.33066907387547E-16));
#17573=DIRECTION('ref_axis',(7.13571935167128E-47,3.33066907387547E-16,
1.));
#17574=DIRECTION('',(9.93056848476794E-32,1.,-3.33066907387547E-16));
#17575=DIRECTION('center_axis',(9.93056848476794E-32,1.,-3.33066907387547E-16));
#17576=DIRECTION('ref_axis',(6.61508746764379E-47,3.33066907387547E-16,
1.));
#17577=DIRECTION('center_axis',(9.93056848476794E-32,1.,-3.33066907387547E-16));
#17578=DIRECTION('ref_axis',(7.13571935167128E-47,3.33066907387547E-16,
1.));
#17579=DIRECTION('center_axis',(9.93056848476794E-32,1.,-3.33066907387547E-16));
#17580=DIRECTION('ref_axis',(7.13571935167128E-47,3.33066907387547E-16,
1.));
#17581=DIRECTION('',(9.93056848476794E-32,1.,-3.33066907387547E-16));
#17582=DIRECTION('center_axis',(9.93056848476794E-32,1.,-3.33066907387547E-16));
#17583=DIRECTION('ref_axis',(6.61508746764379E-47,3.33066907387547E-16,
1.));
#17584=DIRECTION('center_axis',(9.93056848476794E-32,1.,-3.33066907387547E-16));
#17585=DIRECTION('ref_axis',(7.13571935167128E-47,3.33066907387547E-16,
1.));
#17586=DIRECTION('center_axis',(9.93056848476794E-32,1.,-3.33066907387547E-16));
#17587=DIRECTION('ref_axis',(7.13571935167128E-47,3.33066907387547E-16,
1.));
#17588=DIRECTION('',(9.93056848476794E-32,1.,-3.33066907387547E-16));
#17589=DIRECTION('center_axis',(9.93056848476794E-32,1.,-3.33066907387547E-16));
#17590=DIRECTION('ref_axis',(6.61508746764379E-47,3.33066907387547E-16,
1.));
#17591=DIRECTION('center_axis',(9.93056848476794E-32,1.,-3.33066907387547E-16));
#17592=DIRECTION('ref_axis',(7.13571935167128E-47,3.33066907387547E-16,
1.));
#17593=DIRECTION('center_axis',(9.93056848476794E-32,1.,-3.33066907387547E-16));
#17594=DIRECTION('ref_axis',(7.13571935167128E-47,3.33066907387547E-16,
1.));
#17595=DIRECTION('',(9.93056848476794E-32,1.,-3.33066907387547E-16));
#17596=DIRECTION('center_axis',(9.93056848476794E-32,1.,-3.33066907387547E-16));
#17597=DIRECTION('ref_axis',(6.61508746764379E-47,3.33066907387547E-16,
1.));
#17598=DIRECTION('center_axis',(9.93056848476794E-32,1.,-3.33066907387547E-16));
#17599=DIRECTION('ref_axis',(7.13571935167128E-47,3.33066907387547E-16,
1.));
#17600=DIRECTION('center_axis',(9.93056848476794E-32,1.,-3.33066907387547E-16));
#17601=DIRECTION('ref_axis',(7.13571935167128E-47,3.33066907387547E-16,
1.));
#17602=DIRECTION('',(9.93056848476794E-32,1.,-3.33066907387547E-16));
#17603=DIRECTION('center_axis',(9.93056848476794E-32,1.,-3.33066907387547E-16));
#17604=DIRECTION('ref_axis',(6.61508746764379E-47,3.33066907387547E-16,
1.));
#17605=DIRECTION('center_axis',(9.93056848476794E-32,1.,-3.33066907387547E-16));
#17606=DIRECTION('ref_axis',(7.13571935166959E-47,3.33066907387547E-16,
1.));
#17607=DIRECTION('center_axis',(9.93056848476794E-32,1.,-3.33066907387547E-16));
#17608=DIRECTION('ref_axis',(7.13571935166959E-47,3.33066907387547E-16,
1.));
#17609=DIRECTION('',(9.93056848476794E-32,1.,-3.33066907387547E-16));
#17610=DIRECTION('center_axis',(9.93056848476794E-32,1.,-3.33066907387547E-16));
#17611=DIRECTION('ref_axis',(6.61508746764379E-47,3.33066907387547E-16,
1.));
#17612=DIRECTION('center_axis',(9.93056848476794E-32,1.,-3.33066907387547E-16));
#17613=DIRECTION('ref_axis',(7.13571935167128E-47,3.33066907387547E-16,
1.));
#17614=DIRECTION('center_axis',(9.93056848476794E-32,1.,-3.33066907387547E-16));
#17615=DIRECTION('ref_axis',(7.13571935167128E-47,3.33066907387547E-16,
1.));
#17616=DIRECTION('',(9.93056848476794E-32,1.,-3.33066907387547E-16));
#17617=DIRECTION('center_axis',(9.93056848476794E-32,1.,-3.33066907387547E-16));
#17618=DIRECTION('ref_axis',(6.61508746764379E-47,3.33066907387547E-16,
1.));
#17619=DIRECTION('center_axis',(9.93056848476794E-32,1.,-3.33066907387547E-16));
#17620=DIRECTION('ref_axis',(7.13571935167128E-47,3.33066907387547E-16,
1.));
#17621=DIRECTION('center_axis',(9.93056848476794E-32,1.,-3.33066907387547E-16));
#17622=DIRECTION('ref_axis',(7.13571935167128E-47,3.33066907387547E-16,
1.));
#17623=DIRECTION('',(9.93056848476794E-32,1.,-3.33066907387547E-16));
#17624=DIRECTION('center_axis',(9.93056848476794E-32,1.,-3.33066907387547E-16));
#17625=DIRECTION('ref_axis',(6.61508746764379E-47,3.33066907387547E-16,
1.));
#17626=DIRECTION('center_axis',(9.93056848476794E-32,1.,-3.33066907387547E-16));
#17627=DIRECTION('ref_axis',(7.13571935167128E-47,3.33066907387547E-16,
1.));
#17628=DIRECTION('center_axis',(9.93056848476794E-32,1.,-3.33066907387547E-16));
#17629=DIRECTION('ref_axis',(7.13571935167128E-47,3.33066907387547E-16,
1.));
#17630=DIRECTION('',(9.93056848476794E-32,1.,-3.33066907387547E-16));
#17631=DIRECTION('center_axis',(9.93056848476794E-32,1.,-3.33066907387547E-16));
#17632=DIRECTION('ref_axis',(6.61508746764379E-47,3.33066907387547E-16,
1.));
#17633=DIRECTION('center_axis',(9.93056848476794E-32,1.,-3.33066907387547E-16));
#17634=DIRECTION('ref_axis',(7.13571935167128E-47,3.33066907387547E-16,
1.));
#17635=DIRECTION('center_axis',(9.93056848476794E-32,1.,-3.33066907387547E-16));
#17636=DIRECTION('ref_axis',(7.13571935167128E-47,3.33066907387547E-16,
1.));
#17637=DIRECTION('',(9.93056848476794E-32,1.,-3.33066907387547E-16));
#17638=DIRECTION('center_axis',(9.93056848476794E-32,1.,-3.33066907387547E-16));
#17639=DIRECTION('ref_axis',(6.61508746764379E-47,3.33066907387547E-16,
1.));
#17640=DIRECTION('center_axis',(9.93056848476794E-32,1.,-3.33066907387547E-16));
#17641=DIRECTION('ref_axis',(6.64176120743267E-47,3.33066907387547E-16,
1.));
#17642=DIRECTION('center_axis',(9.93056848476794E-32,1.,-3.33066907387547E-16));
#17643=DIRECTION('ref_axis',(6.64176120743267E-47,3.33066907387547E-16,
1.));
#17644=DIRECTION('',(9.93056848476794E-32,1.,-3.33066907387547E-16));
#17645=DIRECTION('center_axis',(9.93056848476794E-32,1.,-3.33066907387547E-16));
#17646=DIRECTION('ref_axis',(6.61508746764379E-47,3.33066907387547E-16,
1.));
#17647=DIRECTION('center_axis',(9.93056848476794E-32,1.,-3.33066907387547E-16));
#17648=DIRECTION('ref_axis',(6.55317088808553E-47,3.33066907387547E-16,
1.));
#17649=DIRECTION('center_axis',(9.93056848476794E-32,1.,-3.33066907387547E-16));
#17650=DIRECTION('ref_axis',(6.55317088808553E-47,3.33066907387547E-16,
1.));
#17651=DIRECTION('',(9.93056848476794E-32,1.,-3.33066907387547E-16));
#17652=DIRECTION('center_axis',(9.93056848476794E-32,1.,-3.33066907387547E-16));
#17653=DIRECTION('ref_axis',(6.61508746764379E-47,3.33066907387547E-16,
1.));
#17654=DIRECTION('center_axis',(9.93056848476794E-32,1.,-3.33066907387547E-16));
#17655=DIRECTION('ref_axis',(7.13571935167128E-47,3.33066907387547E-16,
1.));
#17656=DIRECTION('center_axis',(9.93056848476794E-32,1.,-3.33066907387547E-16));
#17657=DIRECTION('ref_axis',(7.13571935167128E-47,3.33066907387547E-16,
1.));
#17658=DIRECTION('',(9.93056848476794E-32,1.,-3.33066907387547E-16));
#17659=DIRECTION('center_axis',(9.93056848476794E-32,1.,-3.33066907387547E-16));
#17660=DIRECTION('ref_axis',(6.61508746764379E-47,3.33066907387547E-16,
1.));
#17661=DIRECTION('center_axis',(1.,9.93056848476794E-32,1.97215226305253E-31));
#17662=DIRECTION('ref_axis',(1.97215226305253E-31,3.33066907387547E-16,
-1.));
#17663=DIRECTION('',(1.97215226305253E-31,3.33066907387547E-16,-1.));
#17664=DIRECTION('',(9.93056848476794E-32,1.,-3.33066907387547E-16));
#17665=DIRECTION('',(1.97215226305253E-31,3.33066907387547E-16,-1.));
#17666=DIRECTION('',(9.93056848476794E-32,1.,-3.33066907387547E-16));
#17667=DIRECTION('center_axis',(2.2186712959341E-31,-3.33066907387547E-16,
1.));
#17668=DIRECTION('ref_axis',(1.,9.93056848476795E-32,-2.2186712959341E-31));
#17669=DIRECTION('',(1.,9.93056848476795E-32,-2.2186712959341E-31));
#17670=DIRECTION('',(9.93056848476794E-32,1.,-3.33066907387547E-16));
#17671=DIRECTION('',(1.,9.93056848476795E-32,-2.2186712959341E-31));
#17672=DIRECTION('center_axis',(-1.,-9.93056848476794E-32,-1.97215226305253E-31));
#17673=DIRECTION('ref_axis',(-1.97215226305253E-31,-3.33066907387547E-16,
1.));
#17674=DIRECTION('',(-1.97215226305253E-31,-3.33066907387547E-16,1.));
#17675=DIRECTION('',(9.93056848476794E-32,1.,-3.33066907387547E-16));
#17676=DIRECTION('',(-1.97215226305253E-31,-3.33066907387547E-16,1.));
#17677=DIRECTION('center_axis',(-2.2186712959341E-31,3.33066907387547E-16,
-1.));
#17678=DIRECTION('ref_axis',(-1.,-9.93056848476795E-32,2.2186712959341E-31));
#17679=DIRECTION('',(-1.,-9.93056848476795E-32,2.2186712959341E-31));
#17680=DIRECTION('',(-1.,-9.93056848476795E-32,2.2186712959341E-31));
#17681=DIRECTION('center_axis',(-9.93056848476793E-32,-1.,-3.33066907387547E-16));
#17682=DIRECTION('ref_axis',(1.97215226305253E-31,3.33066907387547E-16,
-1.));
#17683=DIRECTION('center_axis',(-9.93056848476793E-32,-1.,-3.33066907387547E-16));
#17684=DIRECTION('ref_axis',(1.97215226305253E-31,3.33066907387547E-16,
-1.));
#17685=DIRECTION('center_axis',(-6.62037898984529E-32,-1.,2.22044604925031E-16));
#17686=DIRECTION('ref_axis',(-2.81594457665554E-47,-2.22044604925031E-16,
-1.));
#17687=DIRECTION('center_axis',(6.62037898984529E-32,1.,-1.60812264967664E-16));
#17688=DIRECTION('ref_axis',(2.94003887450835E-47,1.60812264967664E-16,
1.));
#17689=DIRECTION('',(6.62037898984529E-32,1.,-2.22044604925031E-16));
#17690=DIRECTION('center_axis',(6.62037898984529E-32,1.,-1.60812264967664E-16));
#17691=DIRECTION('ref_axis',(2.41056327970272E-47,1.60812264967664E-16,
1.));
#17692=DIRECTION('center_axis',(-6.62037898984529E-32,-1.,2.22044604925031E-16));
#17693=DIRECTION('ref_axis',(-2.98319463103498E-47,-2.22044604925031E-16,
-1.));
#17694=DIRECTION('center_axis',(6.62037898984529E-32,1.,-1.60812264967664E-16));
#17695=DIRECTION('ref_axis',(2.57781333408216E-47,1.60812264967664E-16,
1.));
#17696=DIRECTION('',(-6.62037898984529E-32,-1.,2.22044604925031E-16));
#17697=DIRECTION('center_axis',(6.62037898984529E-32,1.,-1.60812264967664E-16));
#17698=DIRECTION('ref_axis',(2.94003887450835E-47,1.60812264967664E-16,
1.));
#17699=DIRECTION('center_axis',(6.62037898984529E-32,1.,2.83276944882399E-16));
#17700=DIRECTION('ref_axis',(-1.4791141972894E-31,-2.83276944882399E-16,
1.));
#17701=DIRECTION('center_axis',(6.62037898984529E-32,1.,2.83276944882399E-16));
#17702=DIRECTION('ref_axis',(-1.4791141972894E-31,-2.83276944882399E-16,
1.));
#17703=DIRECTION('center_axis',(5.74253288599218E-16,-1.,2.22044604925031E-16));
#17704=DIRECTION('ref_axis',(1.,5.74253288599218E-16,7.6798984248757E-32));
#17705=DIRECTION('center_axis',(-5.74253288599218E-16,1.,-1.60812264967664E-16));
#17706=DIRECTION('ref_axis',(-1.,-5.74253288599218E-16,1.83632660503434E-32));
#17707=DIRECTION('',(-5.74253288599218E-16,1.,-2.22044604925031E-16));
#17708=DIRECTION('center_axis',(-5.74253288599218E-16,1.,-1.60812264967664E-16));
#17709=DIRECTION('ref_axis',(-1.,-5.74253288599218E-16,-5.56204399040829E-32));
#17710=DIRECTION('center_axis',(5.74253288599218E-16,-1.,2.22044604925031E-16));
#17711=DIRECTION('ref_axis',(1.,5.74253288599218E-16,1.07225475232373E-31));
#17712=DIRECTION('center_axis',(-5.74253288599218E-16,1.,-1.60812264967664E-16));
#17713=DIRECTION('ref_axis',(-1.,-5.74253288599218E-16,-7.76563408967936E-32));
#17714=DIRECTION('',(5.74253288599218E-16,-1.,2.22044604925031E-16));
#17715=DIRECTION('center_axis',(-5.74253288599218E-16,1.,-1.60812264967664E-16));
#17716=DIRECTION('ref_axis',(-1.,-5.74253288599219E-16,7.34531555398823E-33));
#17717=DIRECTION('center_axis',(-5.74253288599219E-16,1.,-1.60812264967664E-16));
#17718=DIRECTION('ref_axis',(-1.,-5.74253288599219E-16,2.95822839457879E-31));
#17719=DIRECTION('center_axis',(-5.74253288599219E-16,1.,-1.60812264967664E-16));
#17720=DIRECTION('ref_axis',(-1.,-5.74253288599219E-16,2.95822839457879E-31));
#17721=DIRECTION('center_axis',(6.62037898984529E-32,1.,-1.60812264967664E-16));
#17722=DIRECTION('ref_axis',(1.06463814030135E-47,1.60812264967664E-16,
1.));
#17723=DIRECTION('center_axis',(6.62037898984529E-32,1.,-1.60812264967664E-16));
#17724=DIRECTION('ref_axis',(1.06463814030135E-47,1.60812264967664E-16,
1.));
#17725=DIRECTION('',(6.62037898984529E-32,1.,-1.60812264967664E-16));
#17726=DIRECTION('center_axis',(6.62037898984529E-32,1.,-1.60812264967664E-16));
#17727=DIRECTION('ref_axis',(1.06463814030135E-47,1.60812264967664E-16,
1.));
#17728=DIRECTION('center_axis',(6.62037898984529E-32,1.,-1.60812264967664E-16));
#17729=DIRECTION('ref_axis',(1.06463814030135E-47,1.60812264967664E-16,
1.));
#17730=DIRECTION('center_axis',(6.62037898984529E-32,1.,-1.60812264967664E-16));
#17731=DIRECTION('ref_axis',(1.06463814030135E-47,1.60812264967664E-16,
1.));
#17732=DIRECTION('',(6.62037898984529E-32,1.,-1.60812264967664E-16));
#17733=DIRECTION('center_axis',(6.62037898984529E-32,1.,-1.60812264967664E-16));
#17734=DIRECTION('ref_axis',(1.06463814030135E-47,1.60812264967664E-16,
1.));
#17735=DIRECTION('center_axis',(6.62037898984529E-32,1.,-1.60812264967664E-16));
#17736=DIRECTION('ref_axis',(1.06463814030135E-47,1.60812264967664E-16,
1.));
#17737=DIRECTION('center_axis',(6.62037898984529E-32,1.,-1.60812264967664E-16));
#17738=DIRECTION('ref_axis',(1.06463814030135E-47,1.60812264967664E-16,
1.));
#17739=DIRECTION('',(6.62037898984529E-32,1.,-1.60812264967664E-16));
#17740=DIRECTION('center_axis',(6.62037898984529E-32,1.,-1.60812264967664E-16));
#17741=DIRECTION('ref_axis',(1.06463814030135E-47,1.60812264967664E-16,
1.));
#17742=DIRECTION('center_axis',(6.62037898984529E-32,1.,-1.60812264967664E-16));
#17743=DIRECTION('ref_axis',(1.06463814030135E-47,1.60812264967664E-16,
1.));
#17744=DIRECTION('center_axis',(6.62037898984529E-32,1.,-1.60812264967664E-16));
#17745=DIRECTION('ref_axis',(1.06463814030135E-47,1.60812264967664E-16,
1.));
#17746=DIRECTION('',(6.62037898984529E-32,1.,-1.60812264967664E-16));
#17747=DIRECTION('center_axis',(6.62037898984529E-32,1.,-1.60812264967664E-16));
#17748=DIRECTION('ref_axis',(1.06463814030135E-47,1.60812264967664E-16,
1.));
#17749=DIRECTION('center_axis',(6.62037898984529E-32,1.,-1.60812264967664E-16));
#17750=DIRECTION('ref_axis',(1.06463814030135E-47,1.60812264967664E-16,
1.));
#17751=DIRECTION('center_axis',(6.62037898984529E-32,1.,-1.60812264967664E-16));
#17752=DIRECTION('ref_axis',(1.06463814030135E-47,1.60812264967664E-16,
1.));
#17753=DIRECTION('',(6.62037898984529E-32,1.,-1.60812264967664E-16));
#17754=DIRECTION('center_axis',(6.62037898984529E-32,1.,-1.60812264967664E-16));
#17755=DIRECTION('ref_axis',(1.06463814030135E-47,1.60812264967664E-16,
1.));
#17756=DIRECTION('center_axis',(6.62037898984529E-32,1.,-1.60812264967664E-16));
#17757=DIRECTION('ref_axis',(1.06463814030135E-47,1.60812264967664E-16,
1.));
#17758=DIRECTION('center_axis',(6.62037898984529E-32,1.,-1.60812264967664E-16));
#17759=DIRECTION('ref_axis',(1.06463814030135E-47,1.60812264967664E-16,
1.));
#17760=DIRECTION('',(6.62037898984529E-32,1.,-1.60812264967664E-16));
#17761=DIRECTION('center_axis',(6.62037898984529E-32,1.,-1.60812264967664E-16));
#17762=DIRECTION('ref_axis',(1.06463814030135E-47,1.60812264967664E-16,
1.));
#17763=DIRECTION('center_axis',(6.62037898984529E-32,1.,-1.60812264967664E-16));
#17764=DIRECTION('ref_axis',(1.06463814030135E-47,1.60812264967664E-16,
1.));
#17765=DIRECTION('center_axis',(6.62037898984529E-32,1.,-1.60812264967664E-16));
#17766=DIRECTION('ref_axis',(1.06463814030135E-47,1.60812264967664E-16,
1.));
#17767=DIRECTION('',(6.62037898984529E-32,1.,-1.60812264967664E-16));
#17768=DIRECTION('center_axis',(6.62037898984529E-32,1.,-1.60812264967664E-16));
#17769=DIRECTION('ref_axis',(1.06463814030135E-47,1.60812264967664E-16,
1.));
#17770=DIRECTION('center_axis',(6.62037898984529E-32,1.,-1.60812264967664E-16));
#17771=DIRECTION('ref_axis',(1.06463814030135E-47,1.60812264967664E-16,
1.));
#17772=DIRECTION('center_axis',(6.62037898984529E-32,1.,-1.60812264967664E-16));
#17773=DIRECTION('ref_axis',(1.06463814030135E-47,1.60812264967664E-16,
1.));
#17774=DIRECTION('',(6.62037898984529E-32,1.,-1.60812264967664E-16));
#17775=DIRECTION('center_axis',(6.62037898984529E-32,1.,-1.60812264967664E-16));
#17776=DIRECTION('ref_axis',(1.06463814030135E-47,1.60812264967664E-16,
1.));
#17777=DIRECTION('center_axis',(6.62037898984529E-32,1.,-1.60812264967664E-16));
#17778=DIRECTION('ref_axis',(1.06463814030135E-47,1.60812264967664E-16,
1.));
#17779=DIRECTION('center_axis',(6.62037898984529E-32,1.,-1.60812264967664E-16));
#17780=DIRECTION('ref_axis',(1.06463814030135E-47,1.60812264967664E-16,
1.));
#17781=DIRECTION('',(6.62037898984529E-32,1.,-1.60812264967664E-16));
#17782=DIRECTION('center_axis',(6.62037898984529E-32,1.,-1.60812264967664E-16));
#17783=DIRECTION('ref_axis',(1.06463814030135E-47,1.60812264967664E-16,
1.));
#17784=DIRECTION('center_axis',(6.62037898984529E-32,1.,-1.60812264967664E-16));
#17785=DIRECTION('ref_axis',(1.06463814030135E-47,1.60812264967664E-16,
1.));
#17786=DIRECTION('center_axis',(6.62037898984529E-32,1.,-1.60812264967664E-16));
#17787=DIRECTION('ref_axis',(1.06463814030135E-47,1.60812264967664E-16,
1.));
#17788=DIRECTION('',(6.62037898984529E-32,1.,-1.60812264967664E-16));
#17789=DIRECTION('center_axis',(6.62037898984529E-32,1.,-1.60812264967664E-16));
#17790=DIRECTION('ref_axis',(1.06463814030135E-47,1.60812264967664E-16,
1.));
#17791=DIRECTION('center_axis',(6.62037898984529E-32,1.,-1.60812264967664E-16));
#17792=DIRECTION('ref_axis',(1.06463814030135E-47,1.60812264967664E-16,
1.));
#17793=DIRECTION('center_axis',(6.62037898984529E-32,1.,-1.60812264967664E-16));
#17794=DIRECTION('ref_axis',(1.06463814030135E-47,1.60812264967664E-16,
1.));
#17795=DIRECTION('',(6.62037898984529E-32,1.,-1.60812264967664E-16));
#17796=DIRECTION('center_axis',(6.62037898984529E-32,1.,-1.60812264967664E-16));
#17797=DIRECTION('ref_axis',(1.06463814030135E-47,1.60812264967664E-16,
1.));
#17798=DIRECTION('center_axis',(6.62037898984529E-32,1.,-1.60812264967664E-16));
#17799=DIRECTION('ref_axis',(1.06463814030135E-47,1.60812264967664E-16,
1.));
#17800=DIRECTION('center_axis',(6.62037898984529E-32,1.,-1.60812264967664E-16));
#17801=DIRECTION('ref_axis',(1.06463814030135E-47,1.60812264967664E-16,
1.));
#17802=DIRECTION('',(6.62037898984529E-32,1.,-1.60812264967664E-16));
#17803=DIRECTION('center_axis',(6.62037898984529E-32,1.,-1.60812264967664E-16));
#17804=DIRECTION('ref_axis',(1.06463814030135E-47,1.60812264967664E-16,
1.));
#17805=DIRECTION('center_axis',(6.62037898984529E-32,1.,-1.60812264967664E-16));
#17806=DIRECTION('ref_axis',(3.06194715830974E-47,1.60812264967664E-16,
1.));
#17807=DIRECTION('center_axis',(6.62037898984529E-32,1.,-1.60812264967664E-16));
#17808=DIRECTION('ref_axis',(3.06194715830974E-47,1.60812264967664E-16,
1.));
#17809=DIRECTION('',(6.62037898984529E-32,1.,-1.60812264967664E-16));
#17810=DIRECTION('center_axis',(6.62037898984529E-32,1.,-1.60812264967664E-16));
#17811=DIRECTION('ref_axis',(2.39617748564028E-47,1.60812264967664E-16,
1.));
#17812=DIRECTION('center_axis',(6.62037898984529E-32,1.,-1.60812264967664E-16));
#17813=DIRECTION('ref_axis',(2.8750069053927E-47,1.60812264967664E-16,1.));
#17814=DIRECTION('center_axis',(6.62037898984529E-32,1.,-1.60812264967664E-16));
#17815=DIRECTION('ref_axis',(2.8750069053927E-47,1.60812264967664E-16,1.));
#17816=DIRECTION('',(-6.62037898984529E-32,-1.,1.60812264967664E-16));
#17817=DIRECTION('center_axis',(6.62037898984529E-32,1.,-1.60812264967664E-16));
#17818=DIRECTION('ref_axis',(2.8750069053927E-47,1.60812264967664E-16,1.));
#17819=DIRECTION('center_axis',(6.62037898984529E-32,1.,2.83276944882399E-16));
#17820=DIRECTION('ref_axis',(-1.4791141972894E-31,-2.83276944882399E-16,
1.));
#17821=DIRECTION('center_axis',(6.62037898984529E-32,1.,2.83276944882399E-16));
#17822=DIRECTION('ref_axis',(-1.4791141972894E-31,-2.83276944882399E-16,
1.));
#17823=DIRECTION('center_axis',(-5.74253288599218E-16,1.,-1.60812264967664E-16));
#17824=DIRECTION('ref_axis',(-1.,-5.74253288599219E-16,9.23469720047697E-32));
#17825=DIRECTION('center_axis',(-5.74253288599218E-16,1.,-1.60812264967664E-16));
#17826=DIRECTION('ref_axis',(-1.,-5.74253288599219E-16,9.23469720047697E-32));
#17827=DIRECTION('',(-5.74253288599219E-16,1.,-1.60812264967664E-16));
#17828=DIRECTION('center_axis',(-5.74253288599218E-16,1.,-1.60812264967664E-16));
#17829=DIRECTION('ref_axis',(-1.,-5.74253288599219E-16,9.23469720047697E-32));
#17830=DIRECTION('center_axis',(-5.74253288599218E-16,1.,-1.60812264967664E-16));
#17831=DIRECTION('ref_axis',(-1.,-5.74253288599219E-16,9.23469720047697E-32));
#17832=DIRECTION('center_axis',(-5.74253288599218E-16,1.,-1.60812264967664E-16));
#17833=DIRECTION('ref_axis',(-1.,-5.74253288599219E-16,9.23469720047697E-32));
#17834=DIRECTION('',(-5.74253288599219E-16,1.,-1.60812264967664E-16));
#17835=DIRECTION('center_axis',(-5.74253288599218E-16,1.,-1.60812264967664E-16));
#17836=DIRECTION('ref_axis',(-1.,-5.74253288599219E-16,9.23469720047697E-32));
#17837=DIRECTION('center_axis',(-5.74253288599218E-16,1.,-1.60812264967664E-16));
#17838=DIRECTION('ref_axis',(-1.,-5.74253288599219E-16,9.23469720047697E-32));
#17839=DIRECTION('center_axis',(-5.74253288599218E-16,1.,-1.60812264967664E-16));
#17840=DIRECTION('ref_axis',(-1.,-5.74253288599219E-16,9.23469720047697E-32));
#17841=DIRECTION('',(-5.74253288599219E-16,1.,-1.60812264967664E-16));
#17842=DIRECTION('center_axis',(-5.74253288599218E-16,1.,-1.60812264967664E-16));
#17843=DIRECTION('ref_axis',(-1.,-5.74253288599219E-16,9.23469720047697E-32));
#17844=DIRECTION('center_axis',(-5.74253288599218E-16,1.,-1.60812264967664E-16));
#17845=DIRECTION('ref_axis',(-1.,-5.74253288599219E-16,9.23469720047697E-32));
#17846=DIRECTION('center_axis',(-5.74253288599218E-16,1.,-1.60812264967664E-16));
#17847=DIRECTION('ref_axis',(-1.,-5.74253288599219E-16,9.23469720047697E-32));
#17848=DIRECTION('',(-5.74253288599219E-16,1.,-1.60812264967664E-16));
#17849=DIRECTION('center_axis',(-5.74253288599218E-16,1.,-1.60812264967664E-16));
#17850=DIRECTION('ref_axis',(-1.,-5.74253288599219E-16,9.23469720047697E-32));
#17851=DIRECTION('center_axis',(-5.74253288599218E-16,1.,-1.60812264967664E-16));
#17852=DIRECTION('ref_axis',(-1.,-5.74253288599219E-16,-5.16348660671831E-32));
#17853=DIRECTION('center_axis',(-5.74253288599218E-16,1.,-1.60812264967664E-16));
#17854=DIRECTION('ref_axis',(-1.,-5.74253288599219E-16,-5.16348660671831E-32));
#17855=DIRECTION('',(-5.74253288599219E-16,1.,-1.60812264967664E-16));
#17856=DIRECTION('center_axis',(-5.74253288599218E-16,1.,-1.60812264967664E-16));
#17857=DIRECTION('ref_axis',(-1.,-5.74253288599219E-16,-5.16348660671831E-32));
#17858=DIRECTION('center_axis',(-5.74253288599218E-16,1.,-1.60812264967664E-16));
#17859=DIRECTION('ref_axis',(-1.,-5.74253288599219E-16,-2.51118958960339E-32));
#17860=DIRECTION('center_axis',(-5.74253288599218E-16,1.,-1.60812264967664E-16));
#17861=DIRECTION('ref_axis',(-1.,-5.74253288599219E-16,-2.51118958960339E-32));
#17862=DIRECTION('',(5.74253288599219E-16,-1.,1.60812264967664E-16));
#17863=DIRECTION('center_axis',(-5.74253288599218E-16,1.,-1.60812264967664E-16));
#17864=DIRECTION('ref_axis',(-1.,-5.74253288599219E-16,-2.51118958960339E-32));
#17865=DIRECTION('center_axis',(-5.74253288599219E-16,1.,-1.60812264967664E-16));
#17866=DIRECTION('ref_axis',(-1.,-5.74253288599219E-16,2.95822839457879E-31));
#17867=DIRECTION('center_axis',(-5.74253288599219E-16,1.,-1.60812264967664E-16));
#17868=DIRECTION('ref_axis',(-1.,-5.74253288599219E-16,2.95822839457879E-31));
#21689=CARTESIAN_POINT('',(0.,0.,0.));
#21690=CARTESIAN_POINT('Origin',(-510.49999999999,-7.9375000000001,442.500000000001));
#21691=CARTESIAN_POINT('',(-510.49999999999,-7.9375000000001,433.500000000001));
#21692=CARTESIAN_POINT('Origin',(-510.49999999999,-7.9375000000001,442.500000000001));
#21693=CARTESIAN_POINT('',(-510.49999999999,-5.88418203051333E-14,433.500000000001));
#21694=CARTESIAN_POINT('',(-510.49999999999,-7.9375000000001,433.500000000001));
#21695=CARTESIAN_POINT('Origin',(-510.49999999999,-5.55111512312578E-14,
442.500000000001));
#21696=CARTESIAN_POINT('Origin',(-510.499999999992,-7.9375000000001,265.5));
#21697=CARTESIAN_POINT('',(-510.499999999992,-7.9375000000001,256.5));
#21698=CARTESIAN_POINT('Origin',(-510.499999999992,-7.9375000000001,265.5));
#21699=CARTESIAN_POINT('',(-510.499999999992,-5.88418203051333E-14,256.5));
#21700=CARTESIAN_POINT('',(-510.499999999992,-7.9375000000001,256.5));
#21701=CARTESIAN_POINT('Origin',(-510.499999999992,-5.55111512312578E-14,
265.5));
#21702=CARTESIAN_POINT('Origin',(-510.499999999994,-7.93750000000004,88.5000000000001));
#21703=CARTESIAN_POINT('',(-510.499999999994,-7.93750000000005,79.5000000000001));
#21704=CARTESIAN_POINT('Origin',(-510.499999999994,-7.93750000000004,88.5000000000001));
#21705=CARTESIAN_POINT('',(-510.499999999994,-3.33066907387547E-15,79.5000000000001));
#21706=CARTESIAN_POINT('',(-510.499999999994,-7.93750000000005,79.5000000000001));
#21707=CARTESIAN_POINT('Origin',(-510.499999999994,0.,88.5000000000001));
#21708=CARTESIAN_POINT('Origin',(-510.499999999996,-7.93750000000004,-88.5));
#21709=CARTESIAN_POINT('',(-510.499999999996,-7.93750000000005,-97.5000000000001));
#21710=CARTESIAN_POINT('Origin',(-510.499999999996,-7.93750000000004,-88.5));
#21711=CARTESIAN_POINT('',(-510.499999999996,-3.33066907387547E-15,-97.5000000000001));
#21712=CARTESIAN_POINT('',(-510.499999999996,-7.93750000000005,-97.5000000000001));
#21713=CARTESIAN_POINT('Origin',(-510.499999999996,0.,-88.5));
#21714=CARTESIAN_POINT('Origin',(-510.499999999998,-7.93749999999999,-265.5));
#21715=CARTESIAN_POINT('',(-510.499999999998,-7.93749999999999,-274.5));
#21716=CARTESIAN_POINT('Origin',(-510.499999999998,-7.93749999999999,-265.5));
#21717=CARTESIAN_POINT('',(-510.499999999998,5.21804821573824E-14,-274.5));
#21718=CARTESIAN_POINT('',(-510.499999999998,-7.93749999999999,-274.5));
#21719=CARTESIAN_POINT('Origin',(-510.499999999998,5.55111512312578E-14,
-265.5));
#21720=CARTESIAN_POINT('Origin',(489.50000000001,-7.9375000000001,442.499999999987));
#21721=CARTESIAN_POINT('',(489.50000000001,-7.9375000000001,433.499999999987));
#21722=CARTESIAN_POINT('Origin',(489.50000000001,-7.9375000000001,442.499999999987));
#21723=CARTESIAN_POINT('',(489.50000000001,-5.88418203051333E-14,433.499999999987));
#21724=CARTESIAN_POINT('',(489.50000000001,-7.9375000000001,433.499999999987));
#21725=CARTESIAN_POINT('Origin',(489.50000000001,-5.55111512312578E-14,
442.499999999987));
#21726=CARTESIAN_POINT('Origin',(289.50000000001,-7.9375000000001,442.49999999999));
#21727=CARTESIAN_POINT('',(289.50000000001,-7.9375000000001,433.499999999989));
#21728=CARTESIAN_POINT('Origin',(289.50000000001,-7.9375000000001,442.49999999999));
#21729=CARTESIAN_POINT('',(289.50000000001,-5.88418203051333E-14,433.499999999989));
#21730=CARTESIAN_POINT('',(289.50000000001,-7.9375000000001,433.499999999989));
#21731=CARTESIAN_POINT('Origin',(289.50000000001,-5.55111512312578E-14,
442.49999999999));
#21732=CARTESIAN_POINT('Origin',(89.5000000000096,-7.9375000000001,442.499999999992));
#21733=CARTESIAN_POINT('',(89.5000000000096,-7.9375000000001,433.499999999992));
#21734=CARTESIAN_POINT('Origin',(89.5000000000096,-7.9375000000001,442.499999999992));
#21735=CARTESIAN_POINT('',(89.5000000000096,-5.88418203051333E-14,433.499999999992));
#21736=CARTESIAN_POINT('',(89.5000000000096,-7.9375000000001,433.499999999992));
#21737=CARTESIAN_POINT('Origin',(89.5000000000096,-5.55111512312578E-14,
442.499999999992));
#21738=CARTESIAN_POINT('Origin',(-110.49999999999,-7.9375000000001,442.499999999995));
#21739=CARTESIAN_POINT('',(-110.49999999999,-7.9375000000001,433.499999999995));
#21740=CARTESIAN_POINT('Origin',(-110.49999999999,-7.9375000000001,442.499999999995));
#21741=CARTESIAN_POINT('',(-110.49999999999,-5.88418203051333E-14,433.499999999995));
#21742=CARTESIAN_POINT('',(-110.49999999999,-7.9375000000001,433.499999999995));
#21743=CARTESIAN_POINT('Origin',(-110.49999999999,-5.55111512312578E-14,
442.499999999995));
#21744=CARTESIAN_POINT('Origin',(-310.499999999991,-7.9375000000001,442.499999999998));
#21745=CARTESIAN_POINT('',(-310.499999999991,-7.9375000000001,433.499999999998));
#21746=CARTESIAN_POINT('Origin',(-310.499999999991,-7.9375000000001,442.499999999998));
#21747=CARTESIAN_POINT('',(-310.499999999991,-5.88418203051333E-14,433.499999999998));
#21748=CARTESIAN_POINT('',(-310.499999999991,-7.9375000000001,433.499999999998));
#21749=CARTESIAN_POINT('Origin',(-310.499999999991,-5.55111512312578E-14,
442.499999999998));
#21750=CARTESIAN_POINT('Origin',(489.500000000001,-7.93749999999999,-442.500000000001));
#21751=CARTESIAN_POINT('',(489.500000000001,-7.93749999999999,-451.500000000005));
#21752=CARTESIAN_POINT('Origin',(489.500000000001,-7.93749999999999,-442.500000000001));
#21753=CARTESIAN_POINT('',(489.500000000001,5.21804821573824E-14,-451.500000000005));
#21754=CARTESIAN_POINT('',(489.500000000001,-7.93749999999999,-451.500000000005));
#21755=CARTESIAN_POINT('Origin',(489.500000000001,5.55111512312578E-14,
-442.500000000001));
#21756=CARTESIAN_POINT('Origin',(289.5,-7.93749999999999,-442.500000000012));
#21757=CARTESIAN_POINT('',(289.5,-7.93749999999999,-451.500000000012));
#21758=CARTESIAN_POINT('Origin',(289.5,-7.93749999999999,-442.500000000012));
#21759=CARTESIAN_POINT('',(289.5,5.21804821573824E-14,-451.500000000012));
#21760=CARTESIAN_POINT('',(289.5,-7.93749999999999,-451.500000000012));
#21761=CARTESIAN_POINT('Origin',(289.5,5.55111512312578E-14,-442.500000000012));
#21762=CARTESIAN_POINT('Origin',(89.5000000000004,-7.93749999999999,-442.500000000009));
#21763=CARTESIAN_POINT('',(89.5000000000004,-7.93749999999999,-451.500000000009));
#21764=CARTESIAN_POINT('Origin',(89.5000000000004,-7.93749999999999,-442.500000000009));
#21765=CARTESIAN_POINT('',(89.5000000000004,5.21804821573824E-14,-451.500000000009));
#21766=CARTESIAN_POINT('',(89.5000000000004,-7.93749999999999,-451.500000000009));
#21767=CARTESIAN_POINT('Origin',(89.5000000000004,5.55111512312578E-14,
-442.500000000009));
#21768=CARTESIAN_POINT('Origin',(-110.5,-7.93749999999999,-442.500000000006));
#21769=CARTESIAN_POINT('',(-110.5,-7.93749999999999,-451.500000000006));
#21770=CARTESIAN_POINT('Origin',(-110.5,-7.93749999999999,-442.500000000006));
#21771=CARTESIAN_POINT('',(-110.5,5.21804821573824E-14,-451.500000000006));
#21772=CARTESIAN_POINT('',(-110.5,-7.93749999999999,-451.500000000006));
#21773=CARTESIAN_POINT('Origin',(-110.5,5.55111512312578E-14,-442.500000000006));
#21774=CARTESIAN_POINT('Origin',(-310.5,-7.93749999999999,-442.500000000003));
#21775=CARTESIAN_POINT('',(-310.5,-7.93749999999999,-451.500000000003));
#21776=CARTESIAN_POINT('Origin',(-310.5,-7.93749999999999,-442.500000000003));
#21777=CARTESIAN_POINT('',(-310.5,5.21804821573824E-14,-451.500000000003));
#21778=CARTESIAN_POINT('',(-310.5,-7.93749999999999,-451.500000000003));
#21779=CARTESIAN_POINT('Origin',(-310.5,5.55111512312578E-14,-442.500000000003));
#21780=CARTESIAN_POINT('Origin',(-278.5,-7.93749999999999,-300.));
#21781=CARTESIAN_POINT('',(-278.5,-7.9375,-331.000000000001));
#21782=CARTESIAN_POINT('Origin',(-278.5,-7.93749999999999,-300.));
#21783=CARTESIAN_POINT('',(-278.5,4.66293670342566E-14,-331.000000000001));
#21784=CARTESIAN_POINT('',(-278.5,-7.9375,-331.000000000001));
#21785=CARTESIAN_POINT('Origin',(-278.5,5.55111512312578E-14,-300.));
#21786=CARTESIAN_POINT('Origin',(-278.5,-7.93750000000004,2.64371857738874E-15));
#21787=CARTESIAN_POINT('',(-278.5,-7.93750000000009,-138.));
#21788=CARTESIAN_POINT('Origin',(-278.5,-7.93750000000004,2.64371857738874E-15));
#21789=CARTESIAN_POINT('',(-278.5,-4.55191440096314E-14,-138.));
#21790=CARTESIAN_POINT('',(-278.5,-7.93750000000009,-138.));
#21791=CARTESIAN_POINT('Origin',(-278.5,0.,7.39557098644699E-29));
#21792=CARTESIAN_POINT('Origin',(-510.5,-7.93749999999999,-442.500000000001));
#21793=CARTESIAN_POINT('',(-510.5,-7.93749999999999,-451.500000000001));
#21794=CARTESIAN_POINT('Origin',(-510.5,-7.93749999999999,-442.500000000001));
#21795=CARTESIAN_POINT('',(-510.5,5.21804821573824E-14,-451.500000000001));
#21796=CARTESIAN_POINT('',(-510.5,-7.93749999999999,-451.500000000001));
#21797=CARTESIAN_POINT('Origin',(-510.5,5.55111512312578E-14,-442.500000000001));
#21798=CARTESIAN_POINT('Origin',(531.5,-7.9375000000001,463.500000000001));
#21799=CARTESIAN_POINT('',(531.5,-5.55111512312578E-14,463.500000000001));
#21800=CARTESIAN_POINT('',(531.5,5.55111512312578E-14,-463.500000000001));
#21801=CARTESIAN_POINT('',(531.5,-5.55111512312578E-14,463.500000000001));
#21802=CARTESIAN_POINT('',(531.5,-7.9375000000001,463.500000000001));
#21803=CARTESIAN_POINT('',(531.5,-7.9375000000001,463.500000000001));
#21804=CARTESIAN_POINT('',(531.5,-7.93749999999999,-463.500000000001));
#21805=CARTESIAN_POINT('',(531.5,-7.9375000000001,463.500000000001));
#21806=CARTESIAN_POINT('',(531.5,-7.93749999999999,-463.500000000001));
#21807=CARTESIAN_POINT('Origin',(-531.5,-7.9375000000001,463.500000000001));
#21808=CARTESIAN_POINT('',(-531.5,-5.55111512312578E-14,463.500000000001));
#21809=CARTESIAN_POINT('',(-531.5,-5.55111512312578E-14,463.500000000001));
#21810=CARTESIAN_POINT('',(-531.5,-7.9375000000001,463.500000000001));
#21811=CARTESIAN_POINT('',(-531.5,-7.9375000000001,463.500000000001));
#21812=CARTESIAN_POINT('',(-531.5,-7.9375000000001,463.500000000001));
#21813=CARTESIAN_POINT('Origin',(-531.5,-7.9375000000001,463.500000000001));
#21814=CARTESIAN_POINT('',(-531.5,5.55111512312578E-14,-463.500000000001));
#21815=CARTESIAN_POINT('',(-531.5,-5.55111512312578E-14,463.500000000001));
#21816=CARTESIAN_POINT('',(-531.5,-7.93749999999999,-463.500000000001));
#21817=CARTESIAN_POINT('',(-531.5,-7.93749999999999,-463.500000000001));
#21818=CARTESIAN_POINT('',(-531.5,-7.9375000000001,463.500000000001));
#21819=CARTESIAN_POINT('Origin',(-531.5,-7.93749999999999,-463.500000000001));
#21820=CARTESIAN_POINT('',(-531.5,5.55111512312578E-14,-463.500000000001));
#21821=CARTESIAN_POINT('',(-531.5,-7.93749999999999,-463.500000000001));
#21822=CARTESIAN_POINT('Origin',(0.,-7.93750000000004,2.6437185773887E-15));
#21823=CARTESIAN_POINT('Origin',(0.,0.,0.));
#21824=CARTESIAN_POINT('Origin',(-278.5,140.,-3.10862446895044E-14));
#21825=CARTESIAN_POINT('',(-278.5,1.77635683940025E-14,136.525));
#21826=CARTESIAN_POINT('Origin',(-278.5,0.,4.93038065763132E-29));
#21827=CARTESIAN_POINT('',(-278.5,140.,136.525));
#21828=CARTESIAN_POINT('',(-278.5,140.,136.525));
#21829=CARTESIAN_POINT('Origin',(-278.5,140.,-3.10862446895044E-14));
#21830=CARTESIAN_POINT('Origin',(-278.5,140.,-3.10862446895044E-14));
#21831=CARTESIAN_POINT('',(-278.5,140.,121.435));
#21832=CARTESIAN_POINT('Origin',(-278.5,140.,-3.10862446895044E-14));
#21833=CARTESIAN_POINT('',(-278.5,0.,121.435));
#21834=CARTESIAN_POINT('',(-278.5,140.,121.435));
#21835=CARTESIAN_POINT('Origin',(-278.5,0.,4.93038065763132E-29));
#21836=CARTESIAN_POINT('Origin',(-278.5,140.,-3.10862446895044E-14));
#21837=CARTESIAN_POINT('Origin',(-278.5,0.,4.93038065763132E-29));
#21838=CARTESIAN_POINT('Origin',(-278.5,232.,-300.));
#21839=CARTESIAN_POINT('',(-308.665,-58.0000000000001,-300.));
#21840=CARTESIAN_POINT('Origin',(-278.5,-58.,-300.));
#21841=CARTESIAN_POINT('',(-308.665,232.,-300.));
#21842=CARTESIAN_POINT('',(-308.665,232.,-300.));
#21843=CARTESIAN_POINT('Origin',(-278.5,232.,-300.));
#21844=CARTESIAN_POINT('Origin',(-278.5,232.,-300.));
#21845=CARTESIAN_POINT('',(-304.755,232.,-300.));
#21846=CARTESIAN_POINT('Origin',(-278.5,232.,-300.));
#21847=CARTESIAN_POINT('',(-304.755,-58.0000000000001,-300.));
#21848=CARTESIAN_POINT('',(-304.755,232.,-300.));
#21849=CARTESIAN_POINT('Origin',(-278.5,-58.,-300.));
#21850=CARTESIAN_POINT('Origin',(-278.5,232.,-300.));
#21851=CARTESIAN_POINT('Origin',(-278.5,-58.,-300.));
#21852=CARTESIAN_POINT('Origin',(-369.,118.3,-156.750598084984));
#21853=CARTESIAN_POINT('',(-369.,118.3,-169.250598084979));
#21854=CARTESIAN_POINT('Origin',(-369.,118.3,-156.750598084984));
#21855=CARTESIAN_POINT('',(-369.,150.,-169.250598084979));
#21856=CARTESIAN_POINT('',(-369.,118.3,-169.250598084979));
#21857=CARTESIAN_POINT('Origin',(-369.,150.,-156.750598084984));
#21858=CARTESIAN_POINT('Origin',(-435.250598084983,118.3,-90.4999999999999));
#21859=CARTESIAN_POINT('',(-435.250598084983,118.3,-102.999999999983));
#21860=CARTESIAN_POINT('Origin',(-435.250598084983,118.3,-90.4999999999999));
#21861=CARTESIAN_POINT('',(-435.250598084983,150.,-102.999999999983));
#21862=CARTESIAN_POINT('',(-435.250598084983,118.3,-102.999999999983));
#21863=CARTESIAN_POINT('Origin',(-435.250598084983,150.,-90.4999999999999));
#21864=CARTESIAN_POINT('Origin',(-459.5,118.3,3.64870602855833E-14));
#21865=CARTESIAN_POINT('',(-459.5,118.3,-12.4999999999698));
#21866=CARTESIAN_POINT('Origin',(-459.5,118.3,3.64870602855833E-14));
#21867=CARTESIAN_POINT('',(-459.5,150.,-12.4999999999698));
#21868=CARTESIAN_POINT('',(-459.5,118.3,-12.4999999999698));
#21869=CARTESIAN_POINT('Origin',(-459.5,150.,3.13893114861083E-14));
#21870=CARTESIAN_POINT('Origin',(-435.250598084983,118.3,90.5000000000001));
#21871=CARTESIAN_POINT('',(-435.250598084983,118.3,78.0000000000418));
#21872=CARTESIAN_POINT('Origin',(-435.250598084983,118.3,90.5000000000001));
#21873=CARTESIAN_POINT('',(-435.250598084983,150.,78.0000000000418));
#21874=CARTESIAN_POINT('',(-435.250598084983,118.3,78.0000000000418));
#21875=CARTESIAN_POINT('Origin',(-435.250598084983,150.,90.5000000000001));
#21876=CARTESIAN_POINT('Origin',(-369.,118.3,156.750598084983));
#21877=CARTESIAN_POINT('',(-369.,118.3,144.250598085032));
#21878=CARTESIAN_POINT('Origin',(-369.,118.3,156.750598084983));
#21879=CARTESIAN_POINT('',(-369.,150.,144.250598085032));
#21880=CARTESIAN_POINT('',(-369.,118.3,144.250598085032));
#21881=CARTESIAN_POINT('Origin',(-369.,150.,156.750598084983));
#21882=CARTESIAN_POINT('Origin',(-278.5,118.3,181.));
#21883=CARTESIAN_POINT('',(-278.5,118.3,168.500000000048));
#21884=CARTESIAN_POINT('Origin',(-278.5,118.3,181.));
#21885=CARTESIAN_POINT('',(-278.5,150.,168.500000000048));
#21886=CARTESIAN_POINT('',(-278.5,118.3,168.500000000048));
#21887=CARTESIAN_POINT('Origin',(-278.5,150.,181.));
#21888=CARTESIAN_POINT('Origin',(-188.,118.3,156.750598084983));
#21889=CARTESIAN_POINT('',(-188.,118.3,144.250598085024));
#21890=CARTESIAN_POINT('Origin',(-188.,118.3,156.750598084983));
#21891=CARTESIAN_POINT('',(-188.,150.,144.250598085024));
#21892=CARTESIAN_POINT('',(-188.,118.3,144.250598085024));
#21893=CARTESIAN_POINT('Origin',(-188.,150.,156.750598084983));
#21894=CARTESIAN_POINT('Origin',(-121.749401915016,118.3,90.5));
#21895=CARTESIAN_POINT('',(-121.749401915016,118.3,78.0000000000295));
#21896=CARTESIAN_POINT('Origin',(-121.749401915016,118.3,90.5));
#21897=CARTESIAN_POINT('',(-121.749401915016,150.,78.0000000000295));
#21898=CARTESIAN_POINT('',(-121.749401915016,118.3,78.0000000000295));
#21899=CARTESIAN_POINT('Origin',(-121.749401915016,150.,90.5));
#21900=CARTESIAN_POINT('Origin',(-97.4999999999999,118.3,-1.90240909456746E-14));
#21901=CARTESIAN_POINT('',(-97.4999999999999,118.3,-12.4999999999835));
#21902=CARTESIAN_POINT('Origin',(-97.4999999999999,118.3,-1.90240909456746E-14));
#21903=CARTESIAN_POINT('',(-97.4999999999999,150.,-12.4999999999835));
#21904=CARTESIAN_POINT('',(-97.4999999999999,118.3,-12.4999999999835));
#21905=CARTESIAN_POINT('Origin',(-97.4999999999999,150.,-2.41218397451495E-14));
#21906=CARTESIAN_POINT('Origin',(-121.749401915016,118.3,-90.5000000000001));
#21907=CARTESIAN_POINT('',(-121.749401915016,118.3,-102.999999999995));
#21908=CARTESIAN_POINT('Origin',(-121.749401915016,118.3,-90.5000000000001));
#21909=CARTESIAN_POINT('',(-121.749401915016,150.,-102.999999999995));
#21910=CARTESIAN_POINT('',(-121.749401915016,118.3,-102.999999999995));
#21911=CARTESIAN_POINT('Origin',(-121.749401915016,150.,-90.5000000000001));
#21912=CARTESIAN_POINT('Origin',(-188.,118.3,-156.750598084983));
#21913=CARTESIAN_POINT('',(-188.,118.3,-169.250598084984));
#21914=CARTESIAN_POINT('Origin',(-188.,118.3,-156.750598084983));
#21915=CARTESIAN_POINT('',(-188.,150.,-169.250598084984));
#21916=CARTESIAN_POINT('',(-188.,118.3,-169.250598084984));
#21917=CARTESIAN_POINT('Origin',(-188.,150.,-156.750598084983));
#21918=CARTESIAN_POINT('Origin',(-278.5,118.3,-181.));
#21919=CARTESIAN_POINT('',(-278.5,118.3,-193.5));
#21920=CARTESIAN_POINT('Origin',(-278.5,118.3,-181.));
#21921=CARTESIAN_POINT('',(-278.5,150.,-193.5));
#21922=CARTESIAN_POINT('',(-278.5,118.3,-193.5));
#21923=CARTESIAN_POINT('Origin',(-278.5,150.,-181.));
#21924=CARTESIAN_POINT('Origin',(-278.5,118.3,-1.90240909456746E-14));
#21925=CARTESIAN_POINT('',(-278.5,118.3,-138.));
#21926=CARTESIAN_POINT('Origin',(-278.5,118.3,-1.90240909456746E-14));
#21927=CARTESIAN_POINT('',(-278.5,150.,-138.));
#21928=CARTESIAN_POINT('',(-278.5,118.3,-138.));
#21929=CARTESIAN_POINT('Origin',(-278.5,150.,-2.41218397451495E-14));
#21930=CARTESIAN_POINT('Origin',(-278.5,118.3,-1.90240909456746E-14));
#21931=CARTESIAN_POINT('',(-278.5,150.,-203.));
#21932=CARTESIAN_POINT('Origin',(-278.5,150.,-2.41218397451495E-14));
#21933=CARTESIAN_POINT('',(-278.5,118.3,-203.));
#21934=CARTESIAN_POINT('',(-278.5,118.3,-203.));
#21935=CARTESIAN_POINT('Origin',(-278.5,118.3,-1.90240909456746E-14));
#21936=CARTESIAN_POINT('Origin',(-278.5,118.3,-1.90240909456746E-14));
#21937=CARTESIAN_POINT('Origin',(-278.5,150.,-2.41218397451495E-14));
#21938=CARTESIAN_POINT('Origin',(-338.999999999999,210.25,-300.));
#21939=CARTESIAN_POINT('',(-329.499999999999,210.25,-300.));
#21940=CARTESIAN_POINT('Origin',(-338.999999999999,210.25,-300.));
#21941=CARTESIAN_POINT('',(-329.499999999999,242.,-300.));
#21942=CARTESIAN_POINT('',(-329.499999999999,210.25,-300.));
#21943=CARTESIAN_POINT('Origin',(-338.999999999999,242.,-300.));
#21944=CARTESIAN_POINT('Origin',(-278.499999999999,210.25,-239.5));
#21945=CARTESIAN_POINT('',(-268.999999999999,210.25,-239.5));
#21946=CARTESIAN_POINT('Origin',(-278.499999999999,210.25,-239.5));
#21947=CARTESIAN_POINT('',(-268.999999999999,242.,-239.5));
#21948=CARTESIAN_POINT('',(-268.999999999999,210.25,-239.5));
#21949=CARTESIAN_POINT('Origin',(-278.499999999999,242.,-239.5));
#21950=CARTESIAN_POINT('Origin',(-217.999999999999,210.25,-300.000000000001));
#21951=CARTESIAN_POINT('',(-208.499999999999,210.25,-300.000000000001));
#21952=CARTESIAN_POINT('Origin',(-217.999999999999,210.25,-300.000000000001));
#21953=CARTESIAN_POINT('',(-208.499999999999,242.,-300.000000000001));
#21954=CARTESIAN_POINT('',(-208.499999999999,210.25,-300.000000000001));
#21955=CARTESIAN_POINT('Origin',(-217.999999999999,242.,-300.000000000001));
#21956=CARTESIAN_POINT('Origin',(-278.5,210.25,-360.5));
#21957=CARTESIAN_POINT('',(-269.,210.25,-360.5));
#21958=CARTESIAN_POINT('Origin',(-278.5,210.25,-360.5));
#21959=CARTESIAN_POINT('',(-269.,242.,-360.5));
#21960=CARTESIAN_POINT('',(-269.,210.25,-360.5));
#21961=CARTESIAN_POINT('Origin',(-278.5,242.,-360.5));
#21962=CARTESIAN_POINT('Origin',(-278.5,210.25,-300.));
#21963=CARTESIAN_POINT('',(-247.5,210.25,-300.));
#21964=CARTESIAN_POINT('Origin',(-278.5,210.25,-300.));
#21965=CARTESIAN_POINT('',(-247.5,242.,-300.));
#21966=CARTESIAN_POINT('',(-247.5,210.25,-300.));
#21967=CARTESIAN_POINT('Origin',(-278.5,242.,-300.));
#21968=CARTESIAN_POINT('Origin',(-278.5,210.25,-300.));
#21969=CARTESIAN_POINT('',(-202.5,242.,-300.));
#21970=CARTESIAN_POINT('Origin',(-278.5,242.,-300.));
#21971=CARTESIAN_POINT('',(-202.5,210.25,-300.));
#21972=CARTESIAN_POINT('',(-202.5,210.25,-300.));
#21973=CARTESIAN_POINT('Origin',(-278.5,210.25,-300.));
#21974=CARTESIAN_POINT('Origin',(-278.5,210.25,-300.));
#21975=CARTESIAN_POINT('Origin',(-278.5,242.,-300.));
#32872=UNCERTAINTY_MEASURE_WITH_UNIT(LENGTH_MEASURE(0.01),#32904,
'DISTANCE_ACCURACY_VALUE',
'Maximum model space distance between geometric entities at asserted c
onnectivities');
#32886=UNCERTAINTY_MEASURE_WITH_UNIT(LENGTH_MEASURE(0.01),#32904,
'DISTANCE_ACCURACY_VALUE',
'Maximum model space distance between geometric entities at asserted c
onnectivities');
#32889=(
GEOMETRIC_REPRESENTATION_CONTEXT(3)
GLOBAL_UNCERTAINTY_ASSIGNED_CONTEXT((#32872))
GLOBAL_UNIT_ASSIGNED_CONTEXT((#32904,#32906,#32907))
REPRESENTATION_CONTEXT('','3D')
);
#32903=(
GEOMETRIC_REPRESENTATION_CONTEXT(3)
GLOBAL_UNCERTAINTY_ASSIGNED_CONTEXT((#32886))
GLOBAL_UNIT_ASSIGNED_CONTEXT((#32904,#32906,#32907))
REPRESENTATION_CONTEXT('','3D')
);
#32904=(
LENGTH_UNIT()
NAMED_UNIT(*)
SI_UNIT(.MILLI.,.METRE.)
);
#32906=(
NAMED_UNIT(*)
PLANE_ANGLE_UNIT()
SI_UNIT($,.RADIAN.)
);
#32907=(
NAMED_UNIT(*)
SI_UNIT($,.STERADIAN.)
SOLID_ANGLE_UNIT()
);
#32910=SHAPE_DEFINITION_REPRESENTATION(#32926,#33014);
#32926=PRODUCT_DEFINITION_SHAPE('',$,#33031);
#33014=SHAPE_REPRESENTATION('',(#15899),#32889);
#33028=PRODUCT_DEFINITION_CONTEXT('part definition',#33078,'design');
#33031=PRODUCT_DEFINITION('Head Cap','Head Cap',#33047,#33028);
#33047=PRODUCT_DEFINITION_FORMATION('',$,#33082);
#33078=APPLICATION_CONTEXT(
'Core Data for Automotive Mechanical Design Process');
#33079=PRODUCT_CONTEXT('part definition',#33078,'mechanical');
#33082=PRODUCT('Head Cap','Head Cap',$,(#33079));
#33097=PRESENTATION_STYLE_ASSIGNMENT((#33103));
#33103=SURFACE_STYLE_USAGE(.BOTH.,#33109);
#33109=SURFACE_SIDE_STYLE('',(#33115));
#33115=SURFACE_STYLE_FILL_AREA(#33121);
#33121=FILL_AREA_STYLE('Opaque(61,176,222)',(#33127));
#33127=FILL_AREA_STYLE_COLOUR('Opaque(61,176,222)',#33133);
#33133=COLOUR_RGB('Opaque(61,176,222)',0.23921568627451,0.690196078431373,
0.870588235294118);
ENDSEC;
END-ISO-10303-21;
